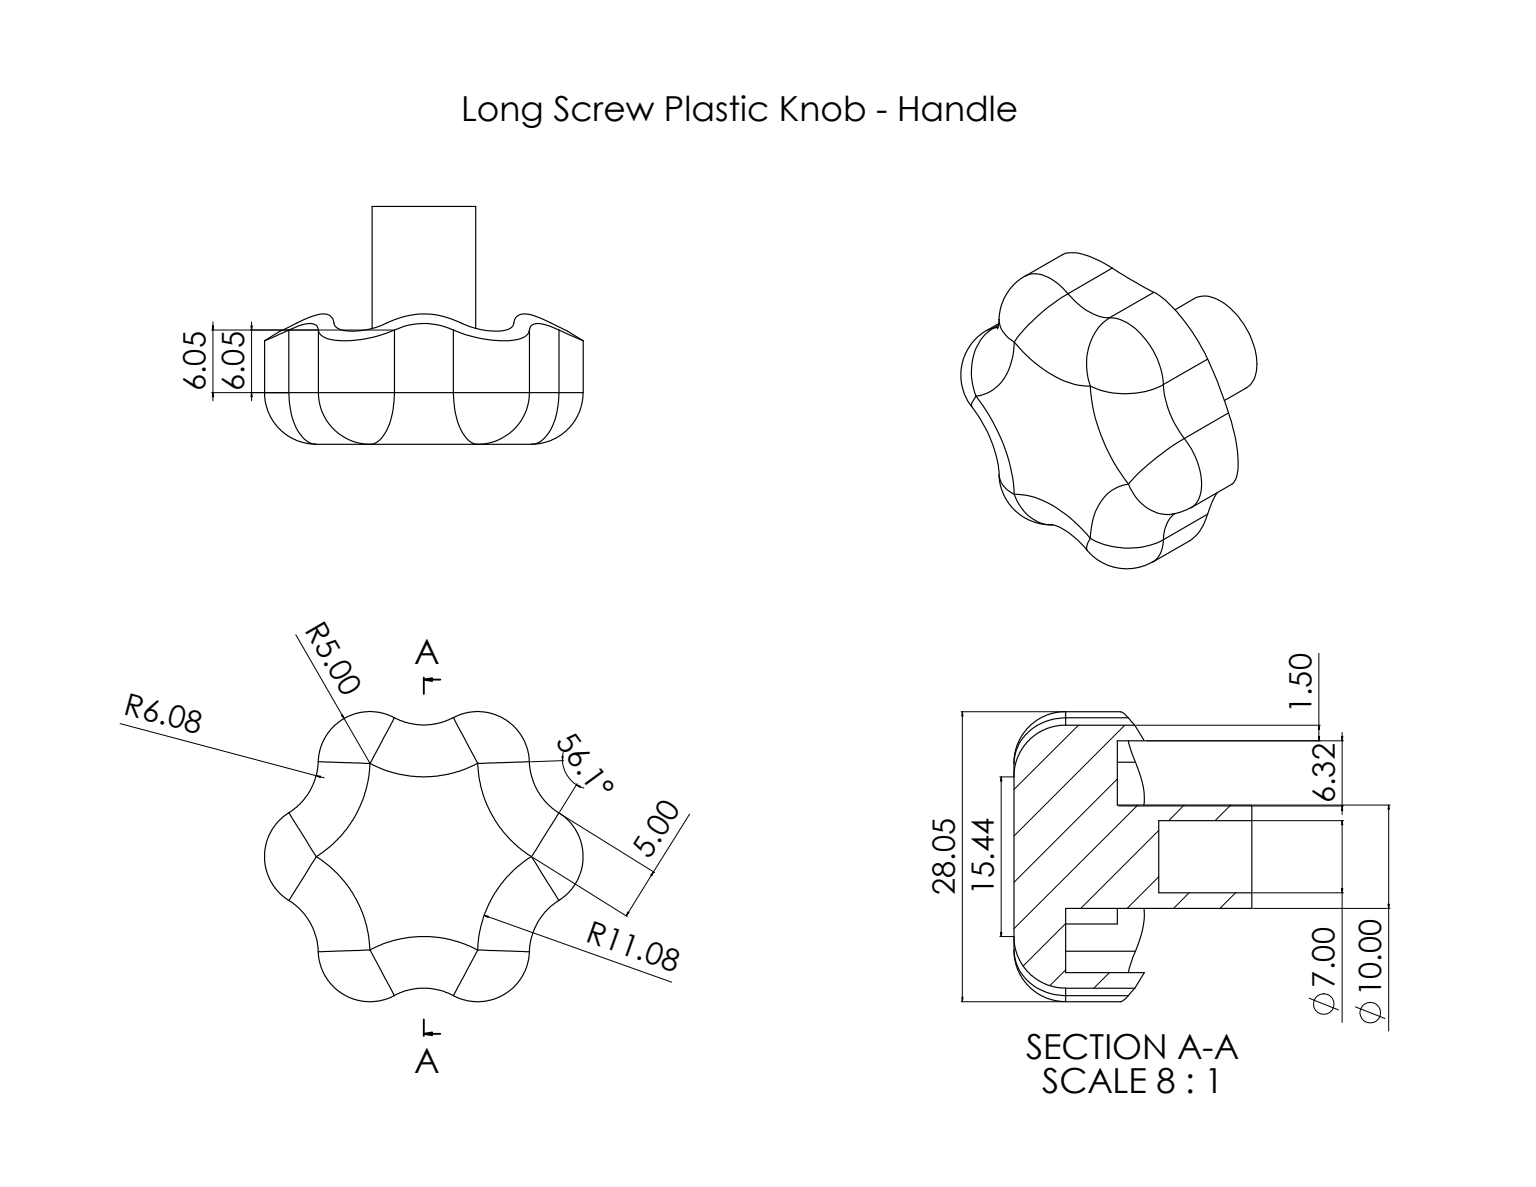
ISO-10303-21;
HEADER;
FILE_DESCRIPTION (('STEP AP214'),
    '1' );
FILE_NAME ('Long Screw Plastic Knob - Handle.step',
    '2026-10-25T21:42:00',
    ( '' ),
    ( '' ),
    'SwSTEP 2.0',
    'SolidWorks 2025',
    '' );
FILE_SCHEMA (( 'AUTOMOTIVE_DESIGN' ));
ENDSEC;

DATA;
#36=CARTESIAN_POINT ( 'NONE',  ( 10.43622283668244677, 12.93305852789453958, 152.0797566693945271 ) ) ;
#58=DIRECTION ( 'NONE',  ( -0.000000000000000000, -0.000000000000000000, -1.000000000000000000 ) ) ;
#59=EDGE_LOOP ( 'NONE', ( #5782, #29938, #317, #14621 ) ) ;
#62=VECTOR ( 'NONE', #37748, 1000.000000000000000 ) ;
#70=DIRECTION ( 'NONE',  ( 0.000000000000000000, 0.000000000000000000, 1.000000000000000000 ) ) ;
#88=CARTESIAN_POINT ( 'NONE',  ( -9.563059451445392156, 11.61997171880338264, 151.9771748954512702 ) ) ;
#133=CARTESIAN_POINT ( 'NONE',  ( -11.30546083962630455, 21.17667637765792676, 152.3877646696492434 ) ) ;
#139=CARTESIAN_POINT ( 'NONE',  ( 12.66061713743917672, 13.00501110736659349, 153.3425884699745723 ) ) ;
#140=CARTESIAN_POINT ( 'NONE',  ( -13.30606428308414380, 19.48475381634399994, 153.3566391844704526 ) ) ;
#160=EDGE_CURVE ( 'NONE', #29981, #18650, #5671, .T. ) ;
#161=CARTESIAN_POINT ( 'NONE',  ( -7.229790860940832786, 5.601750392630878039, 153.6451024802804568 ) ) ;
#162=ORIENTED_EDGE ( 'NONE', *, *, #29231, .F. ) ;
#170=CIRCLE ( 'NONE', #4941, 5.000000000000001776 ) ;
#200=CIRCLE ( 'NONE', #40954, 3.500000000000001332 ) ;
#224=CIRCLE ( 'NONE', #23934, 5.000000000000000888 ) ;
#225=ORIENTED_EDGE ( 'NONE', *, *, #1604, .T. ) ;
#239=CARTESIAN_POINT ( 'NONE',  ( -1.000000000000119460, 22.39897948556632201, 155.5815388724490163 ) ) ;
#242=ADVANCED_FACE ( 'NONE', ( #13025 ), #15594, .T. ) ;
#262=CARTESIAN_POINT ( 'NONE',  ( 12.86284886260855487, 21.86886135845661272, 153.4374325591894603 ) ) ;
#269=DIRECTION ( 'NONE',  ( -0.9994203709764841737, -0.03404294460276034023, 0.000000000000000000 ) ) ;
#299=DIRECTION ( 'NONE',  ( -1.000000000000000000, 0.000000000000000000, 0.000000000000000000 ) ) ;
#311=DIRECTION ( 'NONE',  ( -0.000000000000000000, -0.000000000000000000, -1.000000000000000000 ) ) ;
#313=AXIS2_PLACEMENT_3D ( 'NONE', #32671, #3532, #32264 ) ;
#317=ORIENTED_EDGE ( 'NONE', *, *, #2957, .F. ) ;
#355=CARTESIAN_POINT ( 'NONE',  ( -10.41947860041774199, 17.49999999999951683, 150.5815388724490163 ) ) ;
#361=ORIENTED_EDGE ( 'NONE', *, *, #4016, .F. ) ;
#364=CIRCLE ( 'NONE', #34339, 5.000000000000000888 ) ;
#375=EDGE_CURVE ( 'NONE', #20375, #8168, #5807, .T. ) ;
#378=CARTESIAN_POINT ( 'NONE',  ( -5.521922812467119357, 30.01281927928243221, 153.4949357518731574 ) ) ;
#387=DIRECTION ( 'NONE',  ( 0.000000000000000000, 0.000000000000000000, -1.000000000000000000 ) ) ;
#404=CARTESIAN_POINT ( 'NONE',  ( -5.209739300208506840, 26.52353316214900047, 150.5815388724490163 ) ) ;
#472=ORIENTED_EDGE ( 'NONE', *, *, #35547, .F. ) ;
#481=CARTESIAN_POINT ( 'NONE',  ( -10.21496935922952787, 26.45512302793272497, 153.4374324903474758 ) ) ;
#489=DIRECTION ( 'NONE',  ( -0.000000000000000000, -0.000000000000000000, -1.000000000000000000 ) ) ;
#506=LINE ( 'NONE', #19862, #4090 ) ;
#577=CARTESIAN_POINT ( 'NONE',  ( -2.858598646996059145, 30.93625767528277848, 153.5324451153149710 ) ) ;
#585=CARTESIAN_POINT ( 'NONE',  ( -8.304048588508432971, 28.16586906230009291, 153.3961973886181624 ) ) ;
#594=CARTESIAN_POINT ( 'NONE',  ( -5.000000000000004441, 17.49999999999998934, 159.5815388724490163 ) ) ;
#601=CARTESIAN_POINT ( 'NONE',  ( 3.603329285779394375, 31.27640273042125330, 153.8406024308885947 ) ) ;
#606=CARTESIAN_POINT ( 'NONE',  ( 4.330127018922280691, 15.00000000000012967, 159.5815388724490163 ) ) ;
#610=DIRECTION ( 'NONE',  ( 0.000000000000000000, 0.000000000000000000, -1.000000000000000000 ) ) ;
#624=LINE ( 'NONE', #4028, #9836 ) ;
#640=ORIENTED_EDGE ( 'NONE', *, *, #10319, .F. ) ;
#645=VERTEX_POINT ( 'NONE', #8520 ) ;
#685=EDGE_CURVE ( 'NONE', #37892, #17339, #16571, .T. ) ;
#696=CARTESIAN_POINT ( 'NONE',  ( -11.28839907014780408, 23.42525252760958310, 152.9200731080178457 ) ) ;
#712=EDGE_CURVE ( 'NONE', #26911, #2576, #2299, .T. ) ;
#719=ADVANCED_FACE ( 'NONE', ( #4504 ), #11100, .T. ) ;
#751=ORIENTED_EDGE ( 'NONE', *, *, #36224, .T. ) ;
#782=ADVANCED_FACE ( 'NONE', ( #24490 ), #37459, .T. ) ;
#813=ORIENTED_EDGE ( 'NONE', *, *, #4636, .T. ) ;
#839=CARTESIAN_POINT ( 'NONE',  ( 0.000000000000000000, 17.49999999999998934, 159.5815388724490163 ) ) ;
#841=EDGE_CURVE ( 'NONE', #38078, #4657, #33552, .T. ) ;
#854=CIRCLE ( 'NONE', #40920, 5.000000000000004441 ) ;
#856=ORIENTED_EDGE ( 'NONE', *, *, #19107, .F. ) ;
#859=LINE ( 'NONE', #1078, #3602 ) ;
#908=VECTOR ( 'NONE', #1611, 1000.000000000000000 ) ;
#913=CARTESIAN_POINT ( 'NONE',  ( -10.49927174262155205, 25.01053898198142633, 153.0192155857724572 ) ) ;
#916=CARTESIAN_POINT ( 'NONE',  ( 0.000000000000000000, 17.49999999999998934, 141.5815388724490163 ) ) ;
#919=ORIENTED_EDGE ( 'NONE', *, *, #6532, .F. ) ;
#930=CARTESIAN_POINT ( 'NONE',  ( -1.196959198423996895E-13, 22.49999999999999289, 159.5815388724490163 ) ) ;
#973=DIRECTION ( 'NONE',  ( 1.000000000000000000, 0.000000000000000000, 0.000000000000000000 ) ) ;
#984=DIRECTION ( 'NONE',  ( -0.000000000000000000, -0.000000000000000000, -1.000000000000000000 ) ) ;
#990=LINE ( 'NONE', #39688, #24682 ) ;
#1007=AXIS2_PLACEMENT_3D ( 'NONE', #15270, #22266, #9511 ) ;
#1046=CYLINDRICAL_SURFACE ( 'NONE', #23464, 5.000000000000000000 ) ;
#1050=DIRECTION ( 'NONE',  ( 0.5291922403339774927, -0.8485019580238492010, 0.000000000000000000 ) ) ;
#1078=CARTESIAN_POINT ( 'NONE',  ( 1.000000000000119460, 5.911571776152701574, 154.5815388724490163 ) ) ;
#1114=DIRECTION ( 'NONE',  ( -1.000000000000000000, 0.000000000000000000, 0.000000000000000000 ) ) ;
#1129=AXIS2_PLACEMENT_3D ( 'NONE', #24829, #30991, #12470 ) ;
#1153=CARTESIAN_POINT ( 'NONE',  ( -10.49712838360467160, 9.983023053045442907, 153.0204462789266131 ) ) ;
#1168=VERTEX_POINT ( 'NONE', #3968 ) ;
#1178=CARTESIAN_POINT ( 'NONE',  ( -10.20684115509089729, 26.69374788516367758, 159.5815388724490163 ) ) ;
#1181=CARTESIAN_POINT ( 'NONE',  ( 0.000000000000000000, 17.49999999999956302, 154.9135024962512546 ) ) ;
#1197=DIRECTION ( 'NONE',  ( 0.000000000000000000, 0.000000000000000000, 1.000000000000000000 ) ) ;
#1230=ORIENTED_EDGE ( 'NONE', *, *, #21514, .F. ) ;
#1233=( NAMED_UNIT ( * ) SI_UNIT ( $, .STERADIAN. ) SOLID_ANGLE_UNIT ( ) );
#1237=ORIENTED_EDGE ( 'NONE', *, *, #40727, .F. ) ;
#1247=LINE ( 'NONE', #11028, #6038 ) ;
#1277=EDGE_CURVE ( 'NONE', #3405, #3157, #40350, .T. ) ;
#1315=DIRECTION ( 'NONE',  ( -0.000000000000000000, 0.000000000000000000, 1.000000000000000000 ) ) ;
#1319=CARTESIAN_POINT ( 'NONE',  ( -10.03587323178440194, 23.29421411192350178, 154.5815388724490163 ) ) ;
#1323=ORIENTED_EDGE ( 'NONE', *, *, #13033, .T. ) ;
#1359=CARTESIAN_POINT ( 'NONE',  ( -10.22308315533814316, 8.783078843579193773, 153.3425882844790067 ) ) ;
#1372=CARTESIAN_POINT ( 'NONE',  ( -2.858598646996156400, 4.063742324715559739, 153.5324451153154541 ) ) ;
#1439=FACE_OUTER_BOUND ( 'NONE', #37211, .T. ) ;
#1444=B_SPLINE_CURVE_WITH_KNOTS ( 'NONE', 3,
 ( #38980, #35787, #33219, #36634, #13036, #3662, #29392, #19825, #20048, #10688, #7286, #20256, #23671, #17068, #262, #26227 ),
 .UNSPECIFIED., .F., .F.,
 ( 4, 2, 2, 2, 2, 2, 2, 4 ),
 ( 2.129600427422370939E-07, 0.001523388048537042310, 0.002284975592784182705, 0.003046563137031323316, 0.003808150681278463495, 0.004569738225525604540, 0.005331325769772745152, 0.006092913314019885763 ),
 .UNSPECIFIED. ) ;
#1464=CARTESIAN_POINT ( 'NONE',  ( 10.41947860041720908, 17.49999999999956302, 159.5815388724490163 ) ) ;
#1516=CARTESIAN_POINT ( 'NONE',  ( 5.209739300208926949, 8.476466837849169877, 159.5815388724490163 ) ) ;
#1523=CARTESIAN_POINT ( 'NONE',  ( 16.28249153430138207, 8.099299129593287461, 159.5815388724490163 ) ) ;
#1531=CARTESIAN_POINT ( 'NONE',  ( 7.470466625468908717, 29.21249557649308670, 153.6264001176285205 ) ) ;
#1534=DIRECTION ( 'NONE',  ( -1.000000000000000000, 0.000000000000000000, 0.000000000000000000 ) ) ;
#1542=CARTESIAN_POINT ( 'NONE',  ( 16.28249153430138207, 8.099299129593287461, 154.5815388724490163 ) ) ;
#1575=ORIENTED_EDGE ( 'NONE', *, *, #40939, .T. ) ;
#1592=CARTESIAN_POINT ( 'NONE',  ( 0.000000000000000000, 17.49999999999998934, 159.5815388724490163 ) ) ;
#1604=EDGE_CURVE ( 'NONE', #13562, #20191, #10047, .T. ) ;
#1609=DIRECTION ( 'NONE',  ( -0.000000000000000000, -0.000000000000000000, 1.000000000000000000 ) ) ;
#1611=DIRECTION ( 'NONE',  ( -0.000000000000000000, -0.000000000000000000, -1.000000000000000000 ) ) ;
#1623=VERTEX_POINT ( 'NONE', #13865 ) ;
#1633=ORIENTED_EDGE ( 'NONE', *, *, #40040, .F. ) ;
#1672=ORIENTED_EDGE ( 'NONE', *, *, #15832, .T. ) ;
#1682=CARTESIAN_POINT ( 'NONE',  ( -16.28249153430137497, 8.099299129593275026, 154.5815388724490163 ) ) ;
#1693=EDGE_CURVE ( 'NONE', #14205, #23076, #12143, .T. ) ;
#1698=VECTOR ( 'NONE', #15687, 1000.000000000000000 ) ;
#1716=CONICAL_SURFACE ( 'NONE', #40427, 15.97057991159785217, 1.017022292416746465 ) ;
#1733=CARTESIAN_POINT ( 'NONE',  ( 9.883105000805365137, 22.82715757353904351, 151.9779334031984774 ) ) ;
#1738=CARTESIAN_POINT ( 'NONE',  ( 0.000000000000000000, 36.30140174081339666, 159.5815388724490163 ) ) ;
#1741=ORIENTED_EDGE ( 'NONE', *, *, #40653, .F. ) ;
#1751=EDGE_CURVE ( 'NONE', #7452, #37682, #14909, .T. ) ;
#1771=CARTESIAN_POINT ( 'NONE',  ( 0.000000000000000000, 0.000000000000000000, 150.5815388724490163 ) ) ;
#1772=CARTESIAN_POINT ( 'NONE',  ( -2.858598646996156400, 4.063742324715559739, 153.5324451153154541 ) ) ;
#1780=ORIENTED_EDGE ( 'NONE', *, *, #10909, .T. ) ;
#1782=ADVANCED_FACE ( 'NONE', ( #8938 ), #5025, .T. ) ;
#1785=EDGE_CURVE ( 'NONE', #32027, #13358, #24912, .T. ) ;
#1788=CARTESIAN_POINT ( 'NONE',  ( -1.974753549813219378, 4.453261797671114408, 153.1965160626535578 ) ) ;
#1816=CARTESIAN_POINT ( 'NONE',  ( 3.500000000000003997, 17.49999999999998934, 155.5815388724490163 ) ) ;
#1834=CARTESIAN_POINT ( 'NONE',  ( -15.41947860041774376, 17.49999999999956657, 154.5727510624246293 ) ) ;
#1852=CARTESIAN_POINT ( 'NONE',  ( -14.54815605848680171, 20.32812363823408575, 154.2016373142952830 ) ) ;
#1859=ORIENTED_EDGE ( 'NONE', *, *, #24561, .F. ) ;
#1864=CARTESIAN_POINT ( 'NONE',  ( -9.718734271692440529, 11.88888615205571320, 159.5815388724490163 ) ) ;
#1875=ORIENTED_EDGE ( 'NONE', *, *, #15991, .T. ) ;
#1878=DIRECTION ( 'NONE',  ( 1.000000000000000000, 0.000000000000000000, 0.000000000000000000 ) ) ;
#1899=VERTEX_POINT ( 'NONE', #31694 ) ;
#1910=CARTESIAN_POINT ( 'NONE',  ( 8.534991945851601258, 7.374913356028258704, 153.2263581680556115 ) ) ;
#1929=DIRECTION ( 'NONE',  ( -0.000000000000000000, 0.000000000000000000, 1.000000000000000000 ) ) ;
#1941=CARTESIAN_POINT ( 'NONE',  ( -1.196959198423996895E-13, 29.08842822384727356, 159.5815388724490163 ) ) ;
#1954=ORIENTED_EDGE ( 'NONE', *, *, #1785, .F. ) ;
#1992=ORIENTED_EDGE ( 'NONE', *, *, #19993, .F. ) ;
#2041=VECTOR ( 'NONE', #21924, 1000.000000000000000 ) ;
#2042=ORIENTED_EDGE ( 'NONE', *, *, #16249, .F. ) ;
#2056=DIRECTION ( 'NONE',  ( -0.8660254037844432595, 0.4999999999999919509, 0.000000000000000000 ) ) ;
#2068=DIRECTION ( 'NONE',  ( 0.000000000000000000, 0.000000000000000000, -1.000000000000000000 ) ) ;
#2076=CARTESIAN_POINT ( 'NONE',  ( 0.000000000000000000, 17.49999999999998934, 159.5815388724490163 ) ) ;
#2081=DIRECTION ( 'NONE',  ( -0.8660254037844432595, 0.4999999999999918954, 0.000000000000000000 ) ) ;
#2094=VERTEX_POINT ( 'NONE', #13822 ) ;
#2098=ORIENTED_EDGE ( 'NONE', *, *, #3993, .F. ) ;
#2101=DIRECTION ( 'NONE',  ( 1.000000000000000000, 0.000000000000000000, 0.000000000000000000 ) ) ;
#2105=DIRECTION ( 'NONE',  ( 1.000000000000000000, 3.562084945903540364E-15, 0.000000000000000000 ) ) ;
#2106=ORIENTED_EDGE ( 'NONE', *, *, #16512, .T. ) ;
#2146=ORIENTED_EDGE ( 'NONE', *, *, #27392, .T. ) ;
#2170=AXIS2_PLACEMENT_3D ( 'NONE', #32736, #7869, #33377 ) ;
#2193=EDGE_CURVE ( 'NONE', #15661, #40121, #624, .T. ) ;
#2209=ORIENTED_EDGE ( 'NONE', *, *, #18837, .F. ) ;
#2212=CARTESIAN_POINT ( 'NONE',  ( 12.73537588372913554, 20.13994587915788870, 153.0791759260050355 ) ) ;
#2257=VERTEX_POINT ( 'NONE', #23096 ) ;
#2272=CARTESIAN_POINT ( 'NONE',  ( -14.16111231062272324, 14.17694842453450299, 154.0318591658869138 ) ) ;
#2284=LINE ( 'NONE', #11847, #10538 ) ;
#2299=CIRCLE ( 'NONE', #36958, 7.579174044925481191 ) ;
#2302=CARTESIAN_POINT ( 'NONE',  ( 10.53587323178443569, 12.57181129186098723, 154.5815388724490163 ) ) ;
#2308=EDGE_CURVE ( 'NONE', #10845, #10531, #16114, .T. ) ;
#2311=ADVANCED_FACE ( 'NONE', ( #35660 ), #2322, .T. ) ;
#2322=CONICAL_SURFACE ( 'NONE', #38330, 15.97057991159785217, 1.017022292416746465 ) ;
#2337=CARTESIAN_POINT ( 'NONE',  ( 8.304048588509031603, 6.834130937698395414, 153.3961973886187025 ) ) ;
#2377=ORIENTED_EDGE ( 'NONE', *, *, #32906, .T. ) ;
#2421=ORIENTED_EDGE ( 'NONE', *, *, #34771, .T. ) ;
#2468=ORIENTED_EDGE ( 'NONE', *, *, #13201, .F. ) ;
#2489=VERTEX_POINT ( 'NONE', #29953 ) ;
#2492=FACE_OUTER_BOUND ( 'NONE', #42089, .T. ) ;
#2493=DIRECTION ( 'NONE',  ( -0.000000000000000000, -0.000000000000000000, -1.000000000000000000 ) ) ;
#2515=CARTESIAN_POINT ( 'NONE',  ( -12.27165144158654542, 14.53024314691596963, 152.8454421597759563 ) ) ;
#2523=ORIENTED_EDGE ( 'NONE', *, *, #39714, .T. ) ;
#2564=ORIENTED_EDGE ( 'NONE', *, *, #29829, .F. ) ;
#2576=VERTEX_POINT ( 'NONE', #30380 ) ;
#2578=PLANE ( 'NONE',  #26237 ) ;
#2600=CARTESIAN_POINT ( 'NONE',  ( 15.12727392775252966, 15.80214688207034968, 154.4499356296060739 ) ) ;
#2603=DIRECTION ( 'NONE',  ( 0.8660254037844432595, -0.4999999999999919509, 0.000000000000000000 ) ) ;
#2604=ADVANCED_FACE ( 'NONE', ( #14845 ), #4848, .T. ) ;
#2608=DIRECTION ( 'NONE',  ( 0.000000000000000000, 0.000000000000000000, 1.000000000000000000 ) ) ;
#2631=DIRECTION ( 'NONE',  ( -0.000000000000000000, 0.000000000000000000, 1.000000000000000000 ) ) ;
#2638=CARTESIAN_POINT ( 'NONE',  ( 3.563940842959628874, 29.61244032134256088, 159.5815388724490163 ) ) ;
#2653=ADVANCED_FACE ( 'NONE', ( #37189 ), #6422, .T. ) ;
#2670=CARTESIAN_POINT ( 'NONE',  ( 1.000000000000119460, 12.60102051443365134, 159.5815388724490163 ) ) ;
#2682=VERTEX_POINT ( 'NONE', #7628 ) ;
#2689=CARTESIAN_POINT ( 'NONE',  ( -15.41947860041774909, 17.06357649946066601, 154.5727510624246861 ) ) ;
#2727=CARTESIAN_POINT ( 'NONE',  ( -3.563940842960075184, 5.387559678655594375, 152.8454421597761552 ) ) ;
#2731=CARTESIAN_POINT ( 'NONE',  ( -1.268010732602997237, 6.177570447869829451, 152.0807008677966223 ) ) ;
#2742=ORIENTED_EDGE ( 'NONE', *, *, #13033, .F. ) ;
#2744=EDGE_CURVE ( 'NONE', #41665, #32078, #27610, .T. ) ;
#2754=CIRCLE ( 'NONE', #26549, 4.999999999999999112 ) ;
#2770=DIRECTION ( 'NONE',  ( -0.000000000000000000, -0.000000000000000000, -1.000000000000000000 ) ) ;
#2798=VERTEX_POINT ( 'NONE', #14017 ) ;
#2816=CARTESIAN_POINT ( 'NONE',  ( 15.41947860041720553, 17.06271552903863054, 154.5727510624243166 ) ) ;
#2859=CIRCLE ( 'NONE', #8288, 5.000000000000004441 ) ;
#2880=CIRCLE ( 'NONE', #22575, 5.000000000000004441 ) ;
#2883=AXIS2_PLACEMENT_3D ( 'NONE', #41231, #9102, #22082 ) ;
#2893=ORIENTED_EDGE ( 'NONE', *, *, #6437, .T. ) ;
#2912=UNCERTAINTY_MEASURE_WITH_UNIT (LENGTH_MEASURE( 1.000000000000000082E-05 ), #13359, 'distance_accuracy_value', 'NONE');
#2915=CARTESIAN_POINT ( 'NONE',  ( -9.555006584822248072, 23.39544065986577692, 151.9779333824603214 ) ) ;
#2925=DIRECTION ( 'NONE',  ( 0.000000000000000000, 0.000000000000000000, -1.000000000000000000 ) ) ;
#2941=CARTESIAN_POINT ( 'NONE',  ( -8.654913651898935356, 7.795446523357140833, 153.0774312600626956 ) ) ;
#2943=CARTESIAN_POINT ( 'NONE',  ( -7.786277848952735781, 28.89725529122591041, 153.5727845928841191 ) ) ;
#2955=ORIENTED_EDGE ( 'NONE', *, *, #40653, .T. ) ;
#2956=EDGE_CURVE ( 'NONE', #28523, #29981, #38995, .T. ) ;
#2957=EDGE_CURVE ( 'NONE', #3492, #4147, #19324, .T. ) ;
#2959=CARTESIAN_POINT ( 'NONE',  ( 4.204107165319143746, 31.42570457654730731, 154.0322825799475766 ) ) ;
#2981=ORIENTED_EDGE ( 'NONE', *, *, #25435, .T. ) ;
#2998=ORIENTED_EDGE ( 'NONE', *, *, #30412, .F. ) ;
#3010=ADVANCED_FACE ( 'NONE', ( #25474 ), #9301, .F. ) ;
#3016=CARTESIAN_POINT ( 'NONE',  ( 5.209739300208269697, 26.52353316214887613, 159.5815388724490163 ) ) ;
#3023=CARTESIAN_POINT ( 'NONE',  ( 15.41947860041720908, 17.49999999999956302, 154.5727510624243166 ) ) ;
#3049=FACE_OUTER_BOUND ( 'NONE', #26591, .T. ) ;
#3061=AXIS2_PLACEMENT_3D ( 'NONE', #11887, #24879, #37839 ) ;
#3071=ADVANCED_FACE ( 'NONE', ( #39689 ), #23542, .F. ) ;
#3095=DIRECTION ( 'NONE',  ( -1.000000000000000000, 0.000000000000000000, 0.000000000000000000 ) ) ;
#3112=CARTESIAN_POINT ( 'NONE',  ( -10.41947860041774199, 17.49999999999951683, 159.5815388724490163 ) ) ;
#3129=CARTESIAN_POINT ( 'NONE',  ( -11.07557039803294607, 21.38447842288499601, 152.2937014864026537 ) ) ;
#3156=CARTESIAN_POINT ( 'NONE',  ( -8.536601555666415209, 7.379771219736498189, 153.2247034666974912 ) ) ;
#3157=VERTEX_POINT ( 'NONE', #29905 ) ;
#3205=EDGE_LOOP ( 'NONE', ( #17899, #20292, #4413 ) ) ;
#3241=ORIENTED_EDGE ( 'NONE', *, *, #32380, .F. ) ;
#3257=ORIENTED_EDGE ( 'NONE', *, *, #33128, .T. ) ;
#3259=CARTESIAN_POINT ( 'NONE',  ( 10.41947860041720908, 17.49999999999956302, 159.5815388724490163 ) ) ;
#3286=CARTESIAN_POINT ( 'NONE',  ( -9.173198941869365797, 10.74543714401176864, 152.0797565808659897 ) ) ;
#3338=DIRECTION ( 'NONE',  ( 0.000000000000000000, 0.000000000000000000, 1.000000000000000000 ) ) ;
#3360=CARTESIAN_POINT ( 'NONE',  ( 0.6437596841449632068, 28.74306530438873963, 151.9992204069320962 ) ) ;
#3361=ORIENTED_EDGE ( 'NONE', *, *, #32867, .F. ) ;
#3362=CARTESIAN_POINT ( 'NONE',  ( 13.06543980208692446, 21.74250979011891971, 150.5815388724490163 ) ) ;
#3373=AXIS2_PLACEMENT_3D ( 'NONE', #38028, #27624, #20833 ) ;
#3377=CIRCLE ( 'NONE', #31912, 5.000000000000004441 ) ;
#3379=CARTESIAN_POINT ( 'NONE',  ( 6.938007057734065341, 31.23522659030811610, 154.5496812852157404 ) ) ;
#3387=CARTESIAN_POINT ( 'NONE',  ( -2.858598646996158177, 4.063742324715557963, 159.5815388724490163 ) ) ;
#3405=VERTEX_POINT ( 'NONE', #28327 ) ;
#3429=AXIS2_PLACEMENT_3D ( 'NONE', #31143, #2631, #25401 ) ;
#3432=CARTESIAN_POINT ( 'NONE',  ( 10.64084095417626230, 13.17005021218726135, 152.1397378211943590 ) ) ;
#3452=DIRECTION ( 'NONE',  ( -1.000000000000000000, 0.000000000000000000, 0.000000000000000000 ) ) ;
#3492=VERTEX_POINT ( 'NONE', #6205 ) ;
#3510=DIRECTION ( 'NONE',  ( -0.8660254037844328234, -0.5000000000000101030, 0.000000000000000000 ) ) ;
#3532=DIRECTION ( 'NONE',  ( 0.000000000000000000, 0.000000000000000000, 1.000000000000000000 ) ) ;
#3558=CARTESIAN_POINT ( 'NONE',  ( -5.084889071861075749, 4.975548446798801372, 153.3961973379654182 ) ) ;
#3564=VERTEX_POINT ( 'NONE', #23199 ) ;
#3577=CARTESIAN_POINT ( 'NONE',  ( 2.302507646137074410E-15, -1.301401740813418195, 154.5815388724490163 ) ) ;
#3602=VECTOR ( 'NONE', #36804, 1000.000000000000000 ) ;
#3603=CARTESIAN_POINT ( 'NONE',  ( -2.858598646996059145, 30.93625767528277848, 153.5324451153149710 ) ) ;
#3607=ORIENTED_EDGE ( 'NONE', *, *, #24128, .T. ) ;
#3612=ORIENTED_EDGE ( 'NONE', *, *, #11547, .T. ) ;
#3653=VECTOR ( 'NONE', #14292, 1000.000000000000114 ) ;
#3662=CARTESIAN_POINT ( 'NONE',  ( 10.77561899351920793, 24.31341356600224302, 152.9200730590035846 ) ) ;
#3676=EDGE_CURVE ( 'NONE', #26392, #16970, #31556, .T. ) ;
#3702=ORIENTED_EDGE ( 'NONE', *, *, #27531, .F. ) ;
#3719=AXIS2_PLACEMENT_3D ( 'NONE', #916, #7508, #33021 ) ;
#3720=DIRECTION ( 'NONE',  ( -0.000000000000000000, -0.000000000000000000, -1.000000000000000000 ) ) ;
#3750=CARTESIAN_POINT ( 'NONE',  ( 14.29598715238342699, 20.66495239839645137, 154.0913466422284728 ) ) ;
#3751=CARTESIAN_POINT ( 'NONE',  ( -13.91947860041774021, 17.80787983862214219, 153.6452861111158086 ) ) ;
#3772=ORIENTED_EDGE ( 'NONE', *, *, #11377, .F. ) ;
#3794=CARTESIAN_POINT ( 'NONE',  ( 3.217162522966638960, 31.12730384257888971, 153.6941203706221870 ) ) ;
#3800=DIRECTION ( 'NONE',  ( -0.000000000000000000, -0.000000000000000000, -1.000000000000000000 ) ) ;
#3805=DIRECTION ( 'NONE',  ( 0.000000000000000000, 0.000000000000000000, -1.000000000000000000 ) ) ;
#3835=EDGE_CURVE ( 'NONE', #2257, #6594, #36327, .T. ) ;
#3854=EDGE_CURVE ( 'NONE', #28523, #29783, #34292, .T. ) ;
#3864=CARTESIAN_POINT ( 'NONE',  ( -6.938007057734935756, 3.764773409689712302, 154.5496812852166784 ) ) ;
#3871=CARTESIAN_POINT ( 'NONE',  ( 5.827333669638361968, 29.97187497973753878, 153.5499869721883783 ) ) ;
#3923=CARTESIAN_POINT ( 'NONE',  ( -13.12951721863655585, 15.28026294324127576, 153.2716563237898697 ) ) ;
#3961=CARTESIAN_POINT ( 'NONE',  ( 10.21496935922993288, 8.544876972066248300, 153.4374324903477600 ) ) ;
#3962=LINE ( 'NONE', #13532, #26130 ) ;
#3968=CARTESIAN_POINT ( 'NONE',  ( 9.276117013689805901, 24.01026919326780629, 159.5815388724490163 ) ) ;
#3993=EDGE_CURVE ( 'NONE', #2576, #8117, #12535, .T. ) ;
#4013=DIRECTION ( 'NONE',  ( -1.000000000000000000, 0.000000000000000000, 0.000000000000000000 ) ) ;
#4016=EDGE_CURVE ( 'NONE', #8962, #38078, #35504, .T. ) ;
#4028=CARTESIAN_POINT ( 'NONE',  ( 10.03587323178444279, 11.70578588807654441, 154.5815388724490163 ) ) ;
#4035=ORIENTED_EDGE ( 'NONE', *, *, #32928, .F. ) ;
#4077=DIRECTION ( 'NONE',  ( -0.000000000000000000, -0.000000000000000000, -1.000000000000000000 ) ) ;
#4090=VECTOR ( 'NONE', #39013, 1000.000000000000000 ) ;
#4094=CARTESIAN_POINT ( 'NONE',  ( 3.500000000000003997, 17.49999999999998934, 150.5815388724490163 ) ) ;
#4147=VERTEX_POINT ( 'NONE', #16784 ) ;
#4152=VECTOR ( 'NONE', #15554, 1000.000000000000000 ) ;
#4173=CARTESIAN_POINT ( 'NONE',  ( -4.330127018922262927, 19.99999999999987566, 155.5815388724490163 ) ) ;
#4182=CARTESIAN_POINT ( 'NONE',  ( 5.209739300208269697, 26.52353316214887613, 159.5815388724490163 ) ) ;
#4183=ORIENTED_EDGE ( 'NONE', *, *, #4675, .T. ) ;
#4197=ORIENTED_EDGE ( 'NONE', *, *, #26666, .F. ) ;
#4206=AXIS2_PLACEMENT_3D ( 'NONE', #35238, #36711, #10561 ) ;
#4225=CARTESIAN_POINT ( 'NONE',  ( 5.209739300208926061, 8.476466837849169877, 150.5815388724490163 ) ) ;
#4232=DIRECTION ( 'NONE',  ( 0.5000000000000039968, -0.8660254037844363761, 0.000000000000000000 ) ) ;
#4244=DIRECTION ( 'NONE',  ( -1.000000000000000000, 0.000000000000000000, -0.000000000000000000 ) ) ;
#4245=ORIENTED_EDGE ( 'NONE', *, *, #9976, .T. ) ;
#4247=TOROIDAL_SURFACE ( 'NONE', #23961, 11.07917404492595814, 5.000000000000000000 ) ;
#4252=ORIENTED_EDGE ( 'NONE', *, *, #24650, .T. ) ;
#4257=ADVANCED_FACE ( 'NONE', ( #7212 ), #1046, .T. ) ;
#4262=VERTEX_POINT ( 'NONE', #606 ) ;
#4269=VECTOR ( 'NONE', #37406, 1000.000000000000000 ) ;
#4295=CARTESIAN_POINT ( 'NONE',  ( 10.41947860041720908, 17.49999999999956302, 150.5815388724490163 ) ) ;
#4308=ORIENTED_EDGE ( 'NONE', *, *, #9976, .F. ) ;
#4334=DIRECTION ( 'NONE',  ( -0.000000000000000000, -0.000000000000000000, -1.000000000000000000 ) ) ;
#4336=DIRECTION ( 'NONE',  ( -1.000000000000000000, 0.000000000000000000, 0.000000000000000000 ) ) ;
#4340=ORIENTED_EDGE ( 'NONE', *, *, #40701, .T. ) ;
#4343=AXIS2_PLACEMENT_3D ( 'NONE', #19268, #3720, #25661 ) ;
#4363=DIRECTION ( 'NONE',  ( 0.000000000000000000, 0.000000000000000000, 1.000000000000000000 ) ) ;
#4399=VERTEX_POINT ( 'NONE', #36268 ) ;
#4413=ORIENTED_EDGE ( 'NONE', *, *, #20722, .T. ) ;
#4416=CARTESIAN_POINT ( 'NONE',  ( -8.707710598626182019, 26.64268346825927836, 152.8454421597756436 ) ) ;
#4429=AXIS2_PLACEMENT_3D ( 'NONE', #39570, #7255, #20227 ) ;
#4434=ADVANCED_FACE ( 'NONE', ( #33286 ), #1716, .T. ) ;
#4470=VERTEX_POINT ( 'NONE', #23947 ) ;
#4502=CARTESIAN_POINT ( 'NONE',  ( -4.204107165319530992, 3.574295423450687625, 154.0322825799484008 ) ) ;
#4504=FACE_OUTER_BOUND ( 'NONE', #41210, .T. ) ;
#4507=CARTESIAN_POINT ( 'NONE',  ( 11.77029632476400245, 20.78244114917104568, 152.5896212872837054 ) ) ;
#4508=CARTESIAN_POINT ( 'NONE',  ( 6.697448051447455697, 29.70650749756346798, 153.6454670853904929 ) ) ;
#4520=CARTESIAN_POINT ( 'NONE',  ( -10.89329215898964698, 24.07621678493666906, 152.9047840745570568 ) ) ;
#4522=( GEOMETRIC_REPRESENTATION_CONTEXT ( 3 ) GLOBAL_UNCERTAINTY_ASSIGNED_CONTEXT ( ( #2912 ) ) GLOBAL_UNIT_ASSIGNED_CONTEXT ( ( #13359, #34175, #1233 ) ) REPRESENTATION_CONTEXT ( 'NONE', 'WORKASPACE' ) );
#4556=B_SPLINE_CURVE_WITH_KNOTS ( 'NONE', 3,
 ( #22498, #15712, #2941, #3156, #25706, #6126, #32072, #38879, #18893, #29289, #15930, #16345, #161, #9540, #16146, #29084, #25498, #38669, #12936, #3558, #35482, #19523, #42082, #25916, #9755, #2727 ),
 .UNSPECIFIED., .F., .F.,
 ( 4, 2, 2, 2, 2, 2, 2, 2, 2, 2, 2, 2, 4 ),
 ( 2.152236452720500467E-07, 0.0009105534912597466760, 0.001365722625066985137, 0.001820891758874223706, 0.002276060892681462059, 0.002731230026488700845, 0.003641568294103180153, 0.004551906561717659026, 0.005007075695524905619, 0.005462244829332150477, 0.005917413963139396202, 0.006372583096946641060, 0.007282921364561104755 ),
 .UNSPECIFIED. ) ;
#4557=CARTESIAN_POINT ( 'NONE',  ( -3.500000000000003997, 17.49999999999998934, 150.5815388724490163 ) ) ;
#4585=B_SPLINE_CURVE_WITH_KNOTS ( 'NONE', 3,
 ( #24866, #8682, #30822, #40397, #15294, #3360, #28879, #35266, #32289, #5920, #22291, #38462, #19106, #41876, #12727, #12295 ),
 .UNSPECIFIED., .F., .F.,
 ( 4, 2, 2, 2, 2, 2, 2, 4 ),
 ( 2.442785351375339512E-07, 0.001910986702701202066, 0.002866357914784243080, 0.003821729126867285178, 0.004777100338950327277, 0.005732471551033368508, 0.006687842763116409739, 0.007643213975199451837 ),
 .UNSPECIFIED. ) ;
#4612=FACE_OUTER_BOUND ( 'NONE', #3205, .T. ) ;
#4616=ORIENTED_EDGE ( 'NONE', *, *, #17565, .T. ) ;
#4630=ADVANCED_FACE ( 'NONE', ( #27745 ), #30947, .T. ) ;
#4635=CARTESIAN_POINT ( 'NONE',  ( -4.742640687119331844, 19.08346433899860273, 155.5815388724490163 ) ) ;
#4636=EDGE_CURVE ( 'NONE', #33258, #26911, #21417, .T. ) ;
#4638=LINE ( 'NONE', #17616, #28163 ) ;
#4657=VERTEX_POINT ( 'NONE', #5407 ) ;
#4671=VERTEX_POINT ( 'NONE', #8183 ) ;
#4675=EDGE_CURVE ( 'NONE', #2798, #26392, #41812, .T. ) ;
#4683=ORIENTED_EDGE ( 'NONE', *, *, #34455, .T. ) ;
#4691=DIRECTION ( 'NONE',  ( 1.000000000000000000, 0.000000000000000000, 0.000000000000000000 ) ) ;
#4713=CARTESIAN_POINT ( 'NONE',  ( 8.745125217306711107, 26.05017165142009361, 152.5993402266560679 ) ) ;
#4718=CARTESIAN_POINT ( 'NONE',  ( 8.075457743340587413, 28.53853537488712888, 153.4949358233095325 ) ) ;
#4754=CARTESIAN_POINT ( 'NONE',  ( -10.88765427151144571, 10.91299973181360450, 152.9052493511311468 ) ) ;
#4779=ORIENTED_EDGE ( 'NONE', *, *, #15832, .F. ) ;
#4839=VECTOR ( 'NONE', #20542, 1000.000000000000000 ) ;
#4845=DIRECTION ( 'NONE',  ( -0.8660254037844328234, -0.5000000000000101030, 0.000000000000000000 ) ) ;
#4848=CYLINDRICAL_SURFACE ( 'NONE', #12525, 5.000000000000004441 ) ;
#4862=DIRECTION ( 'NONE',  ( 0.000000000000000000, 1.000000000000000000, 0.000000000000000000 ) ) ;
#4873=ORIENTED_EDGE ( 'NONE', *, *, #13006, .F. ) ;
#4874=CARTESIAN_POINT ( 'NONE',  ( -8.707710598626928089, 8.357316531739311216, 159.5815388724490163 ) ) ;
#4941=AXIS2_PLACEMENT_3D ( 'NONE', #24828, #12251, #25236 ) ;
#4966=DIRECTION ( 'NONE',  ( 0.000000000000000000, 1.000000000000000000, 0.000000000000000000 ) ) ;
#4969=DIRECTION ( 'NONE',  ( 0.000000000000000000, 1.000000000000000000, 0.000000000000000000 ) ) ;
#4973=AXIS2_PLACEMENT_3D ( 'NONE', #8074, #31242, #2105 ) ;
#5025=TOROIDAL_SURFACE ( 'NONE', #10467, 11.07917404492548030, 5.000000000000000000 ) ;
#5032=EDGE_LOOP ( 'NONE', ( #24242, #41500, #5467, #26629 ) ) ;
#5070=VECTOR ( 'NONE', #19222, 1000.000000000000000 ) ;
#5080=ORIENTED_EDGE ( 'NONE', *, *, #15741, .F. ) ;
#5089=CIRCLE ( 'NONE', #7135, 5.000000000000000000 ) ;
#5112=CARTESIAN_POINT ( 'NONE',  ( 11.77722871187724252, 14.20158540853836193, 152.5993403437909706 ) ) ;
#5127=AXIS2_PLACEMENT_3D ( 'NONE', #25479, #12062, #6105 ) ;
#5139=DIRECTION ( 'NONE',  ( -0.000000000000000000, 0.000000000000000000, 1.000000000000000000 ) ) ;
#5140=EDGE_CURVE ( 'NONE', #29783, #20414, #32700, .T. ) ;
#5170=DIRECTION ( 'NONE',  ( -0.000000000000000000, 0.000000000000000000, 1.000000000000000000 ) ) ;
#5183=CARTESIAN_POINT ( 'NONE',  ( 9.535873231784194104, 24.16023951570828032, 154.5815388724490163 ) ) ;
#5184=CARTESIAN_POINT ( 'NONE',  ( 7.326644855052992789, 3.925684524727749647, 154.5725613197538735 ) ) ;
#5194=VERTEX_POINT ( 'NONE', #29291 ) ;
#5235=DIRECTION ( 'NONE',  ( -0.000000000000000000, -0.000000000000000000, 1.000000000000000000 ) ) ;
#5250=EDGE_CURVE ( 'NONE', #10573, #33855, #14011, .T. ) ;
#5252=CARTESIAN_POINT ( 'NONE',  ( 8.707710598626619003, 8.357316531739471088, 159.5815388724490163 ) ) ;
#5262=CARTESIAN_POINT ( 'NONE',  ( -10.27611701369020381, 22.27821838569869684, 159.5815388724490163 ) ) ;
#5266=DIRECTION ( 'NONE',  ( 1.000000000000000000, 0.000000000000000000, 0.000000000000000000 ) ) ;
#5272=LINE ( 'NONE', #18245, #15345 ) ;
#5347=CARTESIAN_POINT ( 'NONE',  ( -1.196959198423996895E-13, 28.72222769588706015, 159.5815388724490163 ) ) ;
#5354=ORIENTED_EDGE ( 'NONE', *, *, #37531, .F. ) ;
#5368=PLANE ( 'NONE',  #26208 ) ;
#5385=CYLINDRICAL_SURFACE ( 'NONE', #41601, 7.579174044924941178 ) ;
#5391=CARTESIAN_POINT ( 'NONE',  ( 2.437533878364066098, 4.288089548799034922, 153.3425884160446913 ) ) ;
#5400=CARTESIAN_POINT ( 'NONE',  ( 13.87973638471548199, 18.10731986427940043, 153.6269493541824431 ) ) ;
#5407=CARTESIAN_POINT ( 'NONE',  ( -5.209739300208506840, 26.52353316214900047, 164.5815388724490163 ) ) ;
#5409=VECTOR ( 'NONE', #70, 1000.000000000000000 ) ;
#5425=CARTESIAN_POINT ( 'NONE',  ( -13.06543980208727618, 21.74250979011898366, 150.5815388724490163 ) ) ;
#5451=VERTEX_POINT ( 'NONE', #41793 ) ;
#5460=CIRCLE ( 'NONE', #12228, 5.000000000000004441 ) ;
#5467=ORIENTED_EDGE ( 'NONE', *, *, #34009, .F. ) ;
#5515=B_SPLINE_CURVE_WITH_KNOTS ( 'NONE', 3,
 ( #25842, #22428, #25635, #6270, #35820, #29213, #35406, #88, #32419, #3286, #32621, #22850, #6681, #32002, #19861, #19652 ),
 .UNSPECIFIED., .F., .F.,
 ( 4, 2, 2, 2, 2, 2, 2, 4 ),
 ( 2.540748634406939408E-07, 0.001910996430635847169, 0.002866367608522052499, 0.003821738786408257395, 0.004777109964294461858, 0.005732481142180667621, 0.006687852320066871650, 0.007643223497953077414 ),
 .UNSPECIFIED. ) ;
#5552=VERTEX_POINT ( 'NONE', #930 ) ;
#5557=DIRECTION ( 'NONE',  ( -1.000000000000000000, 0.000000000000000000, -0.000000000000000000 ) ) ;
#5561=CARTESIAN_POINT ( 'NONE',  ( -2.858598646996159509, 4.063742324715557075, 150.5815388724490163 ) ) ;
#5641=CARTESIAN_POINT ( 'NONE',  ( -9.535873231784242066, 10.83976048429175520, 154.5815388724490163 ) ) ;
#5671=CIRCLE ( 'NONE', #11787, 5.000000000000000000 ) ;
#5676=AXIS2_PLACEMENT_3D ( 'NONE', #1682, #40183, #34015 ) ;
#5699=PLANE ( 'NONE',  #42098 ) ;
#5741=CARTESIAN_POINT ( 'NONE',  ( 7.887293579986041969, 6.217443341193099826, 153.5499870077387357 ) ) ;
#5757=AXIS2_PLACEMENT_3D ( 'NONE', #38059, #38265, #41469 ) ;
#5758=ORIENTED_EDGE ( 'NONE', *, *, #30153, .F. ) ;
#5764=LINE ( 'NONE', #18312, #26384 ) ;
#5778=CARTESIAN_POINT ( 'NONE',  ( 16.28249153430137852, 26.90070087040669122, 159.5815388724490163 ) ) ;
#5779=ADVANCED_FACE ( 'NONE', ( #34507 ), #4247, .T. ) ;
#5782=ORIENTED_EDGE ( 'NONE', *, *, #20269, .F. ) ;
#5785=EDGE_CURVE ( 'NONE', #40356, #29125, #37706, .T. ) ;
#5795=SPHERICAL_SURFACE ( 'NONE', #28267, 5.000000000000000000 ) ;
#5801=ORIENTED_EDGE ( 'NONE', *, *, #15562, .F. ) ;
#5807=LINE ( 'NONE', #22380, #21968 ) ;
#5813=CARTESIAN_POINT ( 'NONE',  ( 5.453575347710441612, 3.477978550085004006, 154.3405383141646610 ) ) ;
#5815=FACE_OUTER_BOUND ( 'NONE', #12151, .T. ) ;
#5846=CARTESIAN_POINT ( 'NONE',  ( 2.302507646137074410E-15, -1.301401740813418195, 159.5815388724490163 ) ) ;
#5863=DIRECTION ( 'NONE',  ( 1.000000000000000000, 0.000000000000000000, 0.000000000000000000 ) ) ;
#5868=DIRECTION ( 'NONE',  ( -0.03404294460293532526, -0.9994203709764784005, -0.000000000000000000 ) ) ;
#5883=CARTESIAN_POINT ( 'NONE',  ( -15.19729569207834885, 16.01032910557492883, 154.4794923609106263 ) ) ;
#5905=CARTESIAN_POINT ( 'NONE',  ( 10.03587323178444279, 11.70578588807654441, 154.5815388724490163 ) ) ;
#5920=CARTESIAN_POINT ( 'NONE',  ( -1.263023857913828651, 28.82150479573344981, 152.0797566321132877 ) ) ;
#5940=DIRECTION ( 'NONE',  ( -0.000000000000000000, -0.000000000000000000, -1.000000000000000000 ) ) ;
#5947=CARTESIAN_POINT ( 'NONE',  ( -3.563940842959833599, 29.61244032134267101, 152.8454421597756152 ) ) ;
#5964=EDGE_CURVE ( 'NONE', #7502, #37842, #13217, .T. ) ;
#6002=SPHERICAL_SURFACE ( 'NONE', #6280, 5.000000000000000000 ) ;
#6010=DIRECTION ( 'NONE',  ( 0.8660254037844363761, 0.5000000000000039968, 0.000000000000000000 ) ) ;
#6012=VECTOR ( 'NONE', #17948, 1000.000000000000000 ) ;
#6013=ORIENTED_EDGE ( 'NONE', *, *, #18837, .T. ) ;
#6032=CARTESIAN_POINT ( 'NONE',  ( -10.53587323178440194, 22.42818870813906429, 154.5815388724490163 ) ) ;
#6038=VECTOR ( 'NONE', #4845, 1000.000000000000000 ) ;
#6085=EDGE_LOOP ( 'NONE', ( #11414, #37575, #17555, #10379, #42068, #16911 ) ) ;
#6102=EDGE_CURVE ( 'NONE', #18422, #40121, #27351, .T. ) ;
#6105=DIRECTION ( 'NONE',  ( 1.000000000000000000, 0.000000000000000000, 0.000000000000000000 ) ) ;
#6120=CARTESIAN_POINT ( 'NONE',  ( -9.276117013690740265, 10.98973080673171765, 154.5815388724490163 ) ) ;
#6123=CARTESIAN_POINT ( 'NONE',  ( 10.27611701369066921, 12.72178161430110066, 154.5815388724490163 ) ) ;
#6126=CARTESIAN_POINT ( 'NONE',  ( -8.372639320098761218, 6.970599522130121350, 153.3561523384327927 ) ) ;
#6127=VERTEX_POINT ( 'NONE', #29366 ) ;
#6128=CARTESIAN_POINT ( 'NONE',  ( -5.970050184154961137, 29.94329617374863517, 153.5717503611250550 ) ) ;
#6129=CARTESIAN_POINT ( 'NONE',  ( 3.563940842959894884, 5.387559678655694739, 152.8454421597760700 ) ) ;
#6138=CARTESIAN_POINT ( 'NONE',  ( 13.12940535518733931, 15.28010775066634608, 153.2716026109635266 ) ) ;
#6161=DIRECTION ( 'NONE',  ( -0.000000000000000000, -0.000000000000000000, -1.000000000000000000 ) ) ;
#6187=AXIS2_PLACEMENT_3D ( 'NONE', #21139, #4969, #17951 ) ;
#6193=EDGE_CURVE ( 'NONE', #7487, #28419, #32984, .T. ) ;
#6205=CARTESIAN_POINT ( 'NONE',  ( 9.718734271691504389, 23.11111384794381252, 154.5815388724490163 ) ) ;
#6214=CARTESIAN_POINT ( 'NONE',  ( 14.54815605848642690, 14.67187636176522858, 154.2016373142949988 ) ) ;
#6236=ADVANCED_FACE ( 'NONE', ( #29793 ), #37036, .T. ) ;
#6249=CARTESIAN_POINT ( 'NONE',  ( 8.707710598625942211, 26.64268346825921085, 152.8454421597755015 ) ) ;
#6250=DIRECTION ( 'NONE',  ( 0.000000000000000000, -0.000000000000000000, -1.000000000000000000 ) ) ;
#6258=CARTESIAN_POINT ( 'NONE',  ( 2.302507646137074410E-15, -1.301401740813418195, 159.5815388724490163 ) ) ;
#6270=CARTESIAN_POINT ( 'NONE',  ( -10.64649782989250504, 13.17637234917139644, 152.1415020206854365 ) ) ;
#6280=AXIS2_PLACEMENT_3D ( 'NONE', #12802, #9408, #38752 ) ;
#6288=ORIENTED_EDGE ( 'NONE', *, *, #6779, .T. ) ;
#6293=VERTEX_POINT ( 'NONE', #23858 ) ;
#6313=CARTESIAN_POINT ( 'NONE',  ( -9.067620284531709984, 24.55832382288969029, 152.1415020426161675 ) ) ;
#6319=CARTESIAN_POINT ( 'NONE',  ( 14.66485744952540315, 20.14980920382255292, 154.2521761610834119 ) ) ;
#6320=CARTESIAN_POINT ( 'NONE',  ( -13.91947860041774376, 17.49999999999951683, 153.6452861111158086 ) ) ;
#6336=CARTESIAN_POINT ( 'NONE',  ( -7.326644855052485639, 31.07431547527046334, 154.5725613197531629 ) ) ;
#6345=AXIS2_PLACEMENT_3D ( 'NONE', #22235, #5235, #18420 ) ;
#6352=CARTESIAN_POINT ( 'NONE',  ( 13.91947860041720908, 17.49999999999956302, 153.6452861111154675 ) ) ;
#6357=CARTESIAN_POINT ( 'NONE',  ( 9.724190303529367085, 28.68314134458470832, 154.2011257354760687 ) ) ;
#6381=CARTESIAN_POINT ( 'NONE',  ( -0.2606827522253820639, 30.22248532900398033, 152.9052493585880086 ) ) ;
#6394=B_SPLINE_CURVE_WITH_KNOTS ( 'NONE', 3,
 ( #16243, #36858, #40249, #17502, #29828, #696, #24102, #4520, #33447, #39392, #913, #36640, #7504, #36204, #481, #23892 ),
 .UNSPECIFIED., .F., .F.,
 ( 4, 2, 2, 2, 2, 2, 2, 4 ),
 ( 2.508354784748761536E-07, 0.001523425935721370523, 0.002285013485842823672, 0.003046601035964277039, 0.003808188586085729972, 0.004569776136207182905, 0.005331363686328636706, 0.006092951236450089639 ),
 .UNSPECIFIED. ) ;
#6422=TOROIDAL_SURFACE ( 'NONE', #7085, 11.07917404492516233, 5.000000000000000000 ) ;
#6433=DIRECTION ( 'NONE',  ( 0.000000000000000000, 0.000000000000000000, -1.000000000000000000 ) ) ;
#6437=EDGE_CURVE ( 'NONE', #4399, #26696, #8869, .T. ) ;
#6438=DIRECTION ( 'NONE',  ( -0.000000000000000000, -0.000000000000000000, -1.000000000000000000 ) ) ;
#6513=EDGE_LOOP ( 'NONE', ( #24766, #35324, #20209 ) ) ;
#6530=DIRECTION ( 'NONE',  ( -1.000000000000000000, 0.000000000000000000, 0.000000000000000000 ) ) ;
#6532=EDGE_CURVE ( 'NONE', #6594, #2798, #25088, .T. ) ;
#6536=CARTESIAN_POINT ( 'NONE',  ( 11.75845712892196637, 12.16770857437972353, 153.0204462570416979 ) ) ;
#6544=VERTEX_POINT ( 'NONE', #28692 ) ;
#6567=CARTESIAN_POINT ( 'NONE',  ( 13.87922053742511075, 16.89024087513384487, 153.6267098343898851 ) ) ;
#6593=CARTESIAN_POINT ( 'NONE',  ( 1.974753549812969577, 30.54673820232729398, 153.1965160626530178 ) ) ;
#6594=VERTEX_POINT ( 'NONE', #3387 ) ;
#6611=ORIENTED_EDGE ( 'NONE', *, *, #27932, .F. ) ;
#6644=CARTESIAN_POINT ( 'NONE',  ( 9.957960250865429686, 6.896283818747226846, 154.0322826691240152 ) ) ;
#6656=AXIS2_PLACEMENT_3D ( 'NONE', #29537, #26359, #10189 ) ;
#6663=LINE ( 'NONE', #19225, #33246 ) ;
#6681=CARTESIAN_POINT ( 'NONE',  ( -8.836825633740376773, 9.547522263686650135, 152.3877645506826468 ) ) ;
#6682=CARTESIAN_POINT ( 'NONE',  ( 0.000000000000000000, 17.49999999999998934, 159.5815388724490163 ) ) ;
#6705=AXIS2_PLACEMENT_3D ( 'NONE', #39600, #32587, #3452 ) ;
#6710=EDGE_LOOP ( 'NONE', ( #29458, #21202, #22666, #38007, #28770, #2893, #12081, #1875, #21194, #4308, #41980, #4873, #16857, #15717, #16433, #41926 ) ) ;
#6714=ADVANCED_FACE ( 'NONE', ( #33798 ), #10619, .F. ) ;
#6730=EDGE_CURVE ( 'NONE', #38421, #37104, #10730, .T. ) ;
#6734=CARTESIAN_POINT ( 'NONE',  ( -12.51134252589945461, 20.32026673028943975, 152.9677466506648784 ) ) ;
#6736=CARTESIAN_POINT ( 'NONE',  ( -5.209739300208506840, 26.52353316214900047, 159.5815388724490163 ) ) ;
#6764=ADVANCED_FACE ( 'NONE', ( #6997 ), #23382, .T. ) ;
#6772=VECTOR ( 'NONE', #39592, 1000.000000000000000 ) ;
#6779=EDGE_CURVE ( 'NONE', #29296, #2682, #12788, .T. ) ;
#6795=CARTESIAN_POINT ( 'NONE',  ( -1.012168522246219782, 30.30180045204023287, 152.9774433921726882 ) ) ;
#6811=ORIENTED_EDGE ( 'NONE', *, *, #11547, .F. ) ;
#6828=CIRCLE ( 'NONE', #11600, 5.000000000000000000 ) ;
#6831=CARTESIAN_POINT ( 'NONE',  ( 8.707710598626619003, 8.357316531739469312, 152.8454421597759847 ) ) ;
#6849=CARTESIAN_POINT ( 'NONE',  ( 9.292375245848642606, 5.582027987049082540, 154.3820435809093397 ) ) ;
#6864=DIRECTION ( 'NONE',  ( 0.000000000000000000, 0.000000000000000000, -1.000000000000000000 ) ) ;
#6896=EDGE_CURVE ( 'NONE', #5451, #17600, #35196, .T. ) ;
#6911=ORIENTED_EDGE ( 'NONE', *, *, #685, .T. ) ;
#6935=CARTESIAN_POINT ( 'NONE',  ( 0.000000000000000000, 17.49999999999998934, 159.5815388724490163 ) ) ;
#6937=FACE_OUTER_BOUND ( 'NONE', #14668, .T. ) ;
#6944=CARTESIAN_POINT ( 'NONE',  ( 13.40983285079566478, 21.52771932643388197, 153.6939610446745519 ) ) ;
#6945=CARTESIAN_POINT ( 'NONE',  ( -13.76218140321603656, 18.54844794216283077, 153.5721917427166829 ) ) ;
#6952=DIRECTION ( 'NONE',  ( -0.000000000000000000, -0.000000000000000000, 1.000000000000000000 ) ) ;
#6962=CARTESIAN_POINT ( 'NONE',  ( -9.411389837926479984, 29.24216370071915705, 154.3424624685361266 ) ) ;
#6976=CARTESIAN_POINT ( 'NONE',  ( 0.000000000000000000, 34.99999999999997868, 154.5815388724490163 ) ) ;
#6980=CIRCLE ( 'NONE', #15788, 7.579174044925158782 ) ;
#6997=FACE_OUTER_BOUND ( 'NONE', #7456, .T. ) ;
#7005=AXIS2_PLACEMENT_3D ( 'NONE', #8058, #36564, #33368 ) ;
#7008=B_SPLINE_CURVE_WITH_KNOTS ( 'NONE', 3,
 ( #32843, #17331, #19665, #13922, #39434, #14134, #27109, #13711, #23282, #3923, #10105, #16698, #20093, #36678 ),
 .UNSPECIFIED., .F., .F.,
 ( 4, 2, 2, 2, 2, 2, 4 ),
 ( 0.003646029068602594809, 0.004555261728908261559, 0.005009878059061094284, 0.005464494389213927876, 0.005919110719366760601, 0.006373727049519594193, 0.007282959709825263979 ),
 .UNSPECIFIED. ) ;
#7011=CARTESIAN_POINT ( 'NONE',  ( 1.254681948488747034, 30.34790559804115873, 153.0192156368753444 ) ) ;
#7038=FACE_OUTER_BOUND ( 'NONE', #34172, .T. ) ;
#7085=AXIS2_PLACEMENT_3D ( 'NONE', #14647, #7848, #5266 ) ;
#7106=DIRECTION ( 'NONE',  ( -1.000000000000000000, 0.000000000000000000, 0.000000000000000000 ) ) ;
#7113=LINE ( 'NONE', #20295, #12992 ) ;
#7128=ORIENTED_EDGE ( 'NONE', *, *, #32380, .T. ) ;
#7135=AXIS2_PLACEMENT_3D ( 'NONE', #8658, #11636, #15268 ) ;
#7163=CARTESIAN_POINT ( 'NONE',  ( 12.28238916904378719, 12.70424003126727541, 153.1863241608643875 ) ) ;
#7164=CARTESIAN_POINT ( 'NONE',  ( -12.73238323000468597, 20.14266894880929115, 153.0776982460621127 ) ) ;
#7166=CYLINDRICAL_SURFACE ( 'NONE', #21429, 3.500000000000001332 ) ;
#7192=EDGE_LOOP ( 'NONE', ( #34117, #24725, #15931, #11677 ) ) ;
#7212=FACE_OUTER_BOUND ( 'NONE', #25185, .T. ) ;
#7229=DIRECTION ( 'NONE',  ( 1.000000000000000000, 0.000000000000000000, 0.000000000000000000 ) ) ;
#7234=AXIS2_PLACEMENT_3D ( 'NONE', #6976, #38675, #35898 ) ;
#7255=DIRECTION ( 'NONE',  ( -0.000000000000000000, 0.000000000000000000, -1.000000000000000000 ) ) ;
#7278=CARTESIAN_POINT ( 'NONE',  ( 5.977173621345689192, 29.94174207387652942, 153.5727845806729022 ) ) ;
#7286=CARTESIAN_POINT ( 'NONE',  ( 11.75395375419299171, 22.83736619992661332, 153.0192156799700172 ) ) ;
#7290=ORIENTED_EDGE ( 'NONE', *, *, #10006, .F. ) ;
#7318=FACE_OUTER_BOUND ( 'NONE', #24148, .T. ) ;
#7394=FACE_OUTER_BOUND ( 'NONE', #22228, .T. ) ;
#7431=DIRECTION ( 'NONE',  ( -1.000000000000000000, 0.000000000000000000, 0.000000000000000000 ) ) ;
#7442=ORIENTED_EDGE ( 'NONE', *, *, #21571, .T. ) ;
#7443=CARTESIAN_POINT ( 'NONE',  ( -2.858598646996059145, 30.93625767528277848, 153.5324451153149710 ) ) ;
#7452=VERTEX_POINT ( 'NONE', #33204 ) ;
#7456=EDGE_LOOP ( 'NONE', ( #4197, #19354, #7806, #24711, #4340, #33162, #11667, #3702 ) ) ;
#7487=VERTEX_POINT ( 'NONE', #4557 ) ;
#7488=CARTESIAN_POINT ( 'NONE',  ( 9.563059451444853920, 23.38002828119538634, 151.9771748954509292 ) ) ;
#7489=CARTESIAN_POINT ( 'NONE',  ( 9.535873231784194104, 24.16023951570828032, 159.5815388724490163 ) ) ;
#7502=VERTEX_POINT ( 'NONE', #25803 ) ;
#7504=CARTESIAN_POINT ( 'NONE',  ( -10.31142999045227704, 25.73355560301168410, 153.1965159924007196 ) ) ;
#7508=DIRECTION ( 'NONE',  ( 0.000000000000000000, 0.000000000000000000, 1.000000000000000000 ) ) ;
#7526=CARTESIAN_POINT ( 'NONE',  ( -8.707710598626182019, 26.64268346825927836, 152.8454421597756436 ) ) ;
#7532=DIRECTION ( 'NONE',  ( 0.5000000000000101030, -0.8660254037844328234, 0.000000000000000000 ) ) ;
#7544=ORIENTED_EDGE ( 'NONE', *, *, #26480, .T. ) ;
#7563=PLANE ( 'NONE',  #36725 ) ;
#7609=CIRCLE ( 'NONE', #13037, 5.000000000000004441 ) ;
#7620=AXIS2_PLACEMENT_3D ( 'NONE', #10838, #4244, #11454 ) ;
#7628=CARTESIAN_POINT ( 'NONE',  ( -4.330127018922124371, 14.99999999999985789, 154.5815388724490163 ) ) ;
#7643=CARTESIAN_POINT ( 'NONE',  ( 10.41947860041720908, 17.49999999999956302, 159.5815388724490163 ) ) ;
#7656=CARTESIAN_POINT ( 'NONE',  ( 0.000000000000000000, 17.49999999999998934, 159.5815388724490163 ) ) ;
#7665=PLANE ( 'NONE',  #26020 ) ;
#7702=LINE ( 'NONE', #7489, #6772 ) ;
#7716=AXIS2_PLACEMENT_3D ( 'NONE', #12512, #9105, #38458 ) ;
#7721=AXIS2_PLACEMENT_3D ( 'NONE', #35970, #36401, #29590 ) ;
#7740=CARTESIAN_POINT ( 'NONE',  ( 13.72762536464759187, 13.72808788916961475, 153.8384576237820909 ) ) ;
#7742=ADVANCED_FACE ( 'NONE', ( #15339 ), #5795, .T. ) ;
#7752=DIRECTION ( 'NONE',  ( -0.000000000000000000, -0.000000000000000000, -1.000000000000000000 ) ) ;
#7760=CARTESIAN_POINT ( 'NONE',  ( -0.2485248900957898466, 4.778023858538846369, 152.9047840822885576 ) ) ;
#7767=ORIENTED_EDGE ( 'NONE', *, *, #41629, .T. ) ;
#7793=EDGE_CURVE ( 'NONE', #8962, #6293, #14372, .T. ) ;
#7806=ORIENTED_EDGE ( 'NONE', *, *, #10006, .T. ) ;
#7821=CIRCLE ( 'NONE', #30242, 5.000000000000004441 ) ;
#7848=DIRECTION ( 'NONE',  ( -0.000000000000000000, 0.000000000000000000, 1.000000000000000000 ) ) ;
#7863=DIRECTION ( 'NONE',  ( 0.000000000000000000, 0.000000000000000000, 1.000000000000000000 ) ) ;
#7869=DIRECTION ( 'NONE',  ( -0.000000000000000000, -0.000000000000000000, -1.000000000000000000 ) ) ;
#7891=CARTESIAN_POINT ( 'NONE',  ( 2.302507646137074410E-15, -1.301401740813418195, 159.5815388724490163 ) ) ;
#7892=DIRECTION ( 'NONE',  ( 0.8660254037844397068, -0.4999999999999979461, 0.000000000000000000 ) ) ;
#7910=DIRECTION ( 'NONE',  ( -0.000000000000000000, -0.000000000000000000, 1.000000000000000000 ) ) ;
#7916=ORIENTED_EDGE ( 'NONE', *, *, #19738, .F. ) ;
#7918=CARTESIAN_POINT ( 'NONE',  ( 8.372639320097622573, 28.02940047786812983, 153.3561523384319401 ) ) ;
#7923=ADVANCED_FACE ( 'NONE', ( #26168 ), #19769, .F. ) ;
#7940=ADVANCED_FACE ( 'NONE', ( #14666 ), #30189, .F. ) ;
#7990=LINE ( 'NONE', #20962, #4839 ) ;
#7991=EDGE_CURVE ( 'NONE', #4671, #12772, #24036, .T. ) ;
#8024=EDGE_LOOP ( 'NONE', ( #1741, #16609, #15313, #20041 ) ) ;
#8048=CARTESIAN_POINT ( 'NONE',  ( -3.742640687119191512, 14.18448485343225585, 154.5815388724490163 ) ) ;
#8058=CARTESIAN_POINT ( 'NONE',  ( 0.000000000000000000, 17.49999999999998934, 159.5815388724490163 ) ) ;
#8059=SPHERICAL_SURFACE ( 'NONE', #26060, 5.000000000000000000 ) ;
#8071=ORIENTED_EDGE ( 'NONE', *, *, #32906, .F. ) ;
#8074=CARTESIAN_POINT ( 'NONE',  ( 2.302507646137074410E-15, -1.301401740813418195, 164.5815388724490163 ) ) ;
#8092=DIRECTION ( 'NONE',  ( 0.000000000000000000, -0.000000000000000000, -1.000000000000000000 ) ) ;
#8109=AXIS2_PLACEMENT_3D ( 'NONE', #41484, #22751, #38278 ) ;
#8117=VERTEX_POINT ( 'NONE', #6123 ) ;
#8163=SPHERICAL_SURFACE ( 'NONE', #6187, 5.000000000000000000 ) ;
#8166=CARTESIAN_POINT ( 'NONE',  ( -2.647879461657173916, 4.176015466079334715, 153.4374325377220885 ) ) ;
#8168=VERTEX_POINT ( 'NONE', #34426 ) ;
#8177=EDGE_CURVE ( 'NONE', #13562, #28722, #16559, .T. ) ;
#8183=CARTESIAN_POINT ( 'NONE',  ( -9.718734271692440529, 11.88888615205571320, 154.5815388724490163 ) ) ;
#8228=AXIS2_PLACEMENT_3D ( 'NONE', #40168, #24429, #27411 ) ;
#8278=VERTEX_POINT ( 'NONE', #2515 ) ;
#8288=AXIS2_PLACEMENT_3D ( 'NONE', #39020, #32227, #3095 ) ;
#8334=AXIS2_PLACEMENT_3D ( 'NONE', #23203, #20443, #14486 ) ;
#8364=CARTESIAN_POINT ( 'NONE',  ( 16.28249153430138207, 8.099299129593287461, 159.5815388724490163 ) ) ;
#8366=CARTESIAN_POINT ( 'NONE',  ( 9.030446397028940808, 5.244147267330249385, 154.4507089031957889 ) ) ;
#8369=AXIS2_PLACEMENT_3D ( 'NONE', #35452, #22689, #23102 ) ;
#8380=ORIENTED_EDGE ( 'NONE', *, *, #23895, .F. ) ;
#8399=VECTOR ( 'NONE', #10882, 1000.000000000000000 ) ;
#8421=ORIENTED_EDGE ( 'NONE', *, *, #39884, .T. ) ;
#8446=EDGE_CURVE ( 'NONE', #8962, #19866, #13391, .T. ) ;
#8464=ORIENTED_EDGE ( 'NONE', *, *, #40413, .F. ) ;
#8478=CARTESIAN_POINT ( 'NONE',  ( -13.06543980208727262, 21.74250979011898721, 153.5324451153151983 ) ) ;
#8517=CARTESIAN_POINT ( 'NONE',  ( 10.41947860041720730, 17.49999999999956302, 164.5815388724490163 ) ) ;
#8520=CARTESIAN_POINT ( 'NONE',  ( -3.563940842960075184, 5.387559678655594375, 152.8454421597761552 ) ) ;
#8540=LINE ( 'NONE', #5561, #31445 ) ;
#8546=CARTESIAN_POINT ( 'NONE',  ( -3.742640687119191512, 14.18448485343225585, 155.5815388724490163 ) ) ;
#8562=ADVANCED_FACE ( 'NONE', ( #4612 ), #34163, .T. ) ;
#8586=CIRCLE ( 'NONE', #1129, 5.000000000000000888 ) ;
#8628=DIRECTION ( 'NONE',  ( -0.000000000000000000, 0.000000000000000000, 1.000000000000000000 ) ) ;
#8642=ORIENTED_EDGE ( 'NONE', *, *, #26666, .T. ) ;
#8658=CARTESIAN_POINT ( 'NONE',  ( -5.209739300209234258, 8.476466837849004676, 159.5815388724490163 ) ) ;
#8682=CARTESIAN_POINT ( 'NONE',  ( 3.042470621311043288, 29.33459613825148438, 152.5896212286789364 ) ) ;
#8691=EDGE_CURVE ( 'NONE', #27377, #36248, #27983, .T. ) ;
#8699=VERTEX_POINT ( 'NONE', #2670 ) ;
#8712=CARTESIAN_POINT ( 'NONE',  ( 5.373768961465674288, 4.977207596738975504, 153.4640811590195426 ) ) ;
#8726=DIRECTION ( 'NONE',  ( 1.000000000000000000, 0.000000000000000000, 0.000000000000000000 ) ) ;
#8733=DIRECTION ( 'NONE',  ( 1.000000000000000000, 0.000000000000000000, 0.000000000000000000 ) ) ;
#8738=CARTESIAN_POINT ( 'NONE',  ( -8.707710598626928089, 8.357316531739311216, 159.5815388724490163 ) ) ;
#8752=ORIENTED_EDGE ( 'NONE', *, *, #18414, .T. ) ;
#8765=B_SPLINE_CURVE_WITH_KNOTS ( 'NONE', 3,
 ( #29268, #6734, #7164, #13755, #39063, #140, #38859, #39694, #39479, #35459, #6945, #25894, #3751, #6320 ),
 .UNSPECIFIED., .F., .F.,
 ( 4, 2, 2, 2, 2, 2, 4 ),
 ( 2.534995934260133079E-07, 0.0009116973918457152134, 0.001367419337971863312, 0.001823141284098011737, 0.002278863230224159944, 0.002734585176350307935, 0.003646029068602594809 ),
 .UNSPECIFIED. ) ;
#8794=PLANE ( 'NONE',  #28590 ) ;
#8798=ORIENTED_EDGE ( 'NONE', *, *, #4636, .F. ) ;
#8803=ORIENTED_EDGE ( 'NONE', *, *, #33688, .T. ) ;
#8811=ORIENTED_EDGE ( 'NONE', *, *, #32189, .F. ) ;
#8844=PRODUCT_DEFINITION ( 'UNKNOWN', '', #36370, #16523 ) ;
#8860=CARTESIAN_POINT ( 'NONE',  ( -14.66485744952595738, 14.85019079617655180, 154.2521761610838666 ) ) ;
#8869=B_SPLINE_CURVE_WITH_KNOTS ( 'NONE', 3,
 ( #15106, #25100, #21686, #18287, #28069, #21481, #31058, #8712, #15324, #41262, #34453, #41049, #11901, #24894, #11483, #38064, #5741, #8922, #14696, #2337, #27860, #40836, #1910, #18086, #11688, #34660 ),
 .UNSPECIFIED., .F., .F.,
 ( 4, 2, 2, 2, 2, 2, 2, 2, 2, 2, 2, 2, 4 ),
 ( 2.437304301980259244E-07, 0.0009105819918573546459, 0.001365751122570934423, 0.001820920253284514199, 0.002276089383998093976, 0.002731258514711673753, 0.003641596776138843281, 0.004551935037566012809, 0.005007104168279592586, 0.005462273298993172363, 0.005917442429706752140, 0.006372611560420331916, 0.007282949821847491470 ),
 .UNSPECIFIED. ) ;
#8883=ORIENTED_EDGE ( 'NONE', *, *, #23219, .T. ) ;
#8903=ORIENTED_EDGE ( 'NONE', *, *, #8446, .F. ) ;
#8907=DIRECTION ( 'NONE',  ( -1.000000000000000000, 0.000000000000000000, 0.000000000000000000 ) ) ;
#8922=CARTESIAN_POINT ( 'NONE',  ( 8.070690082936398113, 6.454723852599054013, 153.4965620064461120 ) ) ;
#8937=ORIENTED_EDGE ( 'NONE', *, *, #5140, .F. ) ;
#8938=FACE_OUTER_BOUND ( 'NONE', #8024, .T. ) ;
#8946=DIRECTION ( 'NONE',  ( -0.000000000000000000, -0.000000000000000000, -1.000000000000000000 ) ) ;
#8962=VERTEX_POINT ( 'NONE', #7443 ) ;
#8982=CARTESIAN_POINT ( 'NONE',  ( 14.29598812252905482, 14.33504584695328532, 154.0913471354969317 ) ) ;
#8985=LINE ( 'NONE', #21958, #23411 ) ;
#9007=VERTEX_POINT ( 'NONE', #26175 ) ;
#9009=CARTESIAN_POINT ( 'NONE',  ( 13.59976475949342678, 18.96908283097675962, 153.4960580910866668 ) ) ;
#9013=FACE_OUTER_BOUND ( 'NONE', #28937, .T. ) ;
#9018=EDGE_CURVE ( 'NONE', #29125, #18650, #224, .T. ) ;
#9069=ORIENTED_EDGE ( 'NONE', *, *, #6779, .F. ) ;
#9081=CARTESIAN_POINT ( 'NONE',  ( -15.41947860041774376, 17.49999999999951683, 150.5815388724490163 ) ) ;
#9096=EDGE_LOOP ( 'NONE', ( #7544, #4616 ) ) ;
#9102=DIRECTION ( 'NONE',  ( -0.000000000000000000, -0.000000000000000000, -1.000000000000000000 ) ) ;
#9105=DIRECTION ( 'NONE',  ( 0.000000000000000000, -0.000000000000000000, -1.000000000000000000 ) ) ;
#9118=VECTOR ( 'NONE', #22891, 1000.000000000000000 ) ;
#9150=VERTEX_POINT ( 'NONE', #23830 ) ;
#9160=VERTEX_POINT ( 'NONE', #8478 ) ;
#9163=AXIS2_PLACEMENT_3D ( 'NONE', #21430, #2068, #31829 ) ;
#9177=VERTEX_POINT ( 'NONE', #4874 ) ;
#9195=ORIENTED_EDGE ( 'NONE', *, *, #6102, .F. ) ;
#9208=EDGE_CURVE ( 'NONE', #35160, #19636, #2880, .T. ) ;
#9229=ADVANCED_FACE ( 'NONE', ( #38671 ), #27356, .T. ) ;
#9232=EDGE_CURVE ( 'NONE', #13300, #26392, #34813, .T. ) ;
#9261=AXIS2_PLACEMENT_3D ( 'NONE', #27595, #30149, #17607 ) ;
#9301=CYLINDRICAL_SURFACE ( 'NONE', #1007, 6.079174044926337395 ) ;
#9324=EDGE_CURVE ( 'NONE', #645, #4399, #38693, .T. ) ;
#9328=CARTESIAN_POINT ( 'NONE',  ( -6.408084924487074119, 29.82586181747419118, 153.6264000693442711 ) ) ;
#9329=CARTESIAN_POINT ( 'NONE',  ( 3.032103446743008579, 5.651413488468350010, 152.5993403105697723 ) ) ;
#9341=ORIENTED_EDGE ( 'NONE', *, *, #31880, .T. ) ;
#9364=EDGE_LOOP ( 'NONE', ( #2468, #1575, #39871, #29144 ) ) ;
#9374=ORIENTED_EDGE ( 'NONE', *, *, #17306, .F. ) ;
#9408=DIRECTION ( 'NONE',  ( 0.000000000000000000, 1.000000000000000000, 0.000000000000000000 ) ) ;
#9409=EDGE_LOOP ( 'NONE', ( #34333, #13294, #17956, #15810 ) ) ;
#9440=VECTOR ( 'NONE', #38897, 1000.000000000000000 ) ;
#9441=CARTESIAN_POINT ( 'NONE',  ( -16.28249153430137497, 8.099299129593275026, 164.5815388724490163 ) ) ;
#9449=DIRECTION ( 'NONE',  ( -0.000000000000000000, 0.000000000000000000, 1.000000000000000000 ) ) ;
#9468=ORIENTED_EDGE ( 'NONE', *, *, #30153, .T. ) ;
#9480=EDGE_LOOP ( 'NONE', ( #38193, #2998, #26283, #21255, #1323, #1633 ) ) ;
#9509=PLANE ( 'NONE',  #8369 ) ;
#9511=DIRECTION ( 'NONE',  ( 1.000000000000000000, 0.000000000000000000, 0.000000000000000000 ) ) ;
#9518=FACE_OUTER_BOUND ( 'NONE', #12461, .T. ) ;
#9531=FACE_OUTER_BOUND ( 'NONE', #15866, .T. ) ;
#9540=CARTESIAN_POINT ( 'NONE',  ( -6.697448051448398054, 5.293492502434390623, 153.6454670853914877 ) ) ;
#9567=AXIS2_PLACEMENT_3D ( 'NONE', #24751, #15392, #15170 ) ;
#9598=AXIS2_PLACEMENT_3D ( 'NONE', #1738, #30665, #8733 ) ;
#9620=DIRECTION ( 'NONE',  ( 1.000000000000000000, 0.000000000000000000, 0.000000000000000000 ) ) ;
#9626=ADVANCED_FACE ( 'NONE', ( #7394 ), #30566, .T. ) ;
#9656=LINE ( 'NONE', #35382, #5070 ) ;
#9689=VECTOR ( 'NONE', #38746, 1000.000000000000000 ) ;
#9723=CARTESIAN_POINT ( 'NONE',  ( 15.97057991159785217, 17.49999999999956302, 154.9135024962512546 ) ) ;
#9729=CARTESIAN_POINT ( 'NONE',  ( -11.77722871187752141, 20.79841459146082272, 152.5993403437912264 ) ) ;
#9735=CARTESIAN_POINT ( 'NONE',  ( 14.54810494377324481, 20.32819496402379045, 154.2016150273000221 ) ) ;
#9736=DIRECTION ( 'NONE',  ( -0.000000000000000000, -0.000000000000000000, -1.000000000000000000 ) ) ;
#9751=CARTESIAN_POINT ( 'NONE',  ( -9.626159306788924397, 28.87726500155387299, 154.2527048017821301 ) ) ;
#9755=CARTESIAN_POINT ( 'NONE',  ( -3.813105931423857342, 5.254802202609886841, 152.9676766465817934 ) ) ;
#9757=ORIENTED_EDGE ( 'NONE', *, *, #9018, .F. ) ;
#9759=AXIS2_PLACEMENT_3D ( 'NONE', #30703, #4334, #33253 ) ;
#9762=AXIS2_PLACEMENT_3D ( 'NONE', #16959, #17176, #30136 ) ;
#9763=ORIENTED_EDGE ( 'NONE', *, *, #15991, .F. ) ;
#9765=PLANE ( 'NONE',  #7234 ) ;
#9776=CARTESIAN_POINT ( 'NONE',  ( 10.13050606591841607, 27.50172420044922106, 153.8381732780032110 ) ) ;
#9786=CARTESIAN_POINT ( 'NONE',  ( 0.000000000000000000, 17.49999999999998934, 154.5815388724490163 ) ) ;
#9806=CARTESIAN_POINT ( 'NONE',  ( -13.91947860041774376, 17.49999999999951683, 159.5815388724490163 ) ) ;
#9810=DIRECTION ( 'NONE',  ( -0.000000000000000000, -0.000000000000000000, -1.000000000000000000 ) ) ;
#9816=VERTEX_POINT ( 'NONE', #1772 ) ;
#9836=VECTOR ( 'NONE', #39975, 1000.000000000000000 ) ;
#9865=CYLINDRICAL_SURFACE ( 'NONE', #38748, 7.579174044925959919 ) ;
#9870=LINE ( 'NONE', #6032, #30618 ) ;
#9918=LINE ( 'NONE', #13302, #16490 ) ;
#9934=DIRECTION ( 'NONE',  ( 1.000000000000000000, 0.000000000000000000, 0.000000000000000000 ) ) ;
#9946=CARTESIAN_POINT ( 'NONE',  ( 10.77809958360015941, 10.69197809562609791, 152.9195735126126010 ) ) ;
#9957=FACE_OUTER_BOUND ( 'NONE', #11940, .T. ) ;
#9973=CARTESIAN_POINT ( 'NONE',  ( 13.30606428308370681, 15.51524618365521491, 153.3566391844701968 ) ) ;
#9976=EDGE_CURVE ( 'NONE', #31801, #10531, #20925, .T. ) ;
#10004=CARTESIAN_POINT ( 'NONE',  ( 5.209739300208273249, 26.52353316214887968, 159.5815388724490163 ) ) ;
#10006=EDGE_CURVE ( 'NONE', #20375, #37916, #6980, .T. ) ;
#10007=ORIENTED_EDGE ( 'NONE', *, *, #16166, .T. ) ;
#10021=ORIENTED_EDGE ( 'NONE', *, *, #9208, .T. ) ;
#10047=LINE ( 'NONE', #1319, #3653 ) ;
#10059=ADVANCED_FACE ( 'NONE', ( #18559 ), #6002, .T. ) ;
#10105=CARTESIAN_POINT ( 'NONE',  ( -13.03525533431007588, 15.17011036820110981, 153.2259575457069616 ) ) ;
#10113=ORIENTED_EDGE ( 'NONE', *, *, #37103, .F. ) ;
#10133=DIRECTION ( 'NONE',  ( 0.000000000000000000, 0.000000000000000000, -1.000000000000000000 ) ) ;
#10141=LINE ( 'NONE', #10353, #36313 ) ;
#10181=CARTESIAN_POINT ( 'NONE',  ( 9.298205070445279219, 29.40977417358551094, 154.3802602823905659 ) ) ;
#10189=DIRECTION ( 'NONE',  ( -1.000000000000000000, 0.000000000000000000, 0.000000000000000000 ) ) ;
#10203=ADVANCED_BREP_SHAPE_REPRESENTATION ( '', ( #36847, #40442 ), #38405 ) ;
#10204=CARTESIAN_POINT ( 'NONE',  ( 2.647879461656943434, 30.82398453391898485, 153.4374325377216621 ) ) ;
#10212=ORIENTED_EDGE ( 'NONE', *, *, #6730, .T. ) ;
#10230=CARTESIAN_POINT ( 'NONE',  ( -1.000000000000119460, 22.39897948556632201, 159.5815388724490163 ) ) ;
#10235=CIRCLE ( 'NONE', #21114, 11.07917404492633828 ) ;
#10261=EDGE_CURVE ( 'NONE', #13719, #19636, #29371, .T. ) ;
#10275=LINE ( 'NONE', #13258, #38024 ) ;
#10319=EDGE_CURVE ( 'NONE', #26696, #11650, #25522, .T. ) ;
#10353=CARTESIAN_POINT ( 'NONE',  ( 1.196959198423996895E-13, 12.49999999999998401, 155.5815388724490163 ) ) ;
#10355=DIRECTION ( 'NONE',  ( -1.000000000000000000, 0.000000000000000000, 0.000000000000000000 ) ) ;
#10360=ORIENTED_EDGE ( 'NONE', *, *, #28217, .T. ) ;
#10379=ORIENTED_EDGE ( 'NONE', *, *, #23944, .T. ) ;
#10396=CARTESIAN_POINT ( 'NONE',  ( 5.039920647268460563, 31.52513099133343033, 154.2527047512469380 ) ) ;
#10461=CARTESIAN_POINT ( 'NONE',  ( -4.408685582965315319, 3.536562997622931803, 154.0918074332477374 ) ) ;
#10466=CARTESIAN_POINT ( 'NONE',  ( 6.417378831301363107, 29.82262957917540191, 153.6272566164921614 ) ) ;
#10467=AXIS2_PLACEMENT_3D ( 'NONE', #37666, #1929, #11501 ) ;
#10480=LINE ( 'NONE', #27071, #40289 ) ;
#10531=VERTEX_POINT ( 'NONE', #22529 ) ;
#10538=VECTOR ( 'NONE', #34820, 1000.000000000000000 ) ;
#10556=AXIS2_PLACEMENT_3D ( 'NONE', #34343, #14784, #37743 ) ;
#10561=DIRECTION ( 'NONE',  ( 1.000000000000000000, 0.000000000000000000, 0.000000000000000000 ) ) ;
#10567=LINE ( 'NONE', #29699, #24097 ) ;
#10573=VERTEX_POINT ( 'NONE', #5947 ) ;
#10599=EDGE_CURVE ( 'NONE', #37941, #9007, #18290, .T. ) ;
#10617=DIRECTION ( 'NONE',  ( -0.8485019580238489789, -0.5291922403339777148, 0.000000000000000000 ) ) ;
#10619=CYLINDRICAL_SURFACE ( 'NONE', #24345, 3.500000000000001332 ) ;
#10622=ORIENTED_EDGE ( 'NONE', *, *, #37881, .T. ) ;
#10637=EDGE_LOOP ( 'NONE', ( #640, #40758, #30457, #2042, #18121, #2098, #33182, #17805 ) ) ;
#10675=CARTESIAN_POINT ( 'NONE',  ( -8.892120608939249493, 5.087317773340616966, 154.4788437280937501 ) ) ;
#10679=CARTESIAN_POINT ( 'NONE',  ( 9.418615391892931399, 23.67094981841350076, 151.9983627776726109 ) ) ;
#10680=FACE_OUTER_BOUND ( 'NONE', #31045, .T. ) ;
#10687=ORIENTED_EDGE ( 'NONE', *, *, #8446, .T. ) ;
#10688=CARTESIAN_POINT ( 'NONE',  ( 11.59049936059900432, 23.02700438487111967, 152.9768715818104852 ) ) ;
#10692=ORIENTED_EDGE ( 'NONE', *, *, #41629, .F. ) ;
#10730=CIRCLE ( 'NONE', #6656, 7.579174044925959919 ) ;
#10736=VERTEX_POINT ( 'NONE', #19977 ) ;
#10785=PLANE ( 'NONE',  #33954 ) ;
#10794=ORIENTED_EDGE ( 'NONE', *, *, #15211, .F. ) ;
#10814=DIRECTION ( 'NONE',  ( -0.000000000000000000, -0.000000000000000000, -1.000000000000000000 ) ) ;
#10832=CARTESIAN_POINT ( 'NONE',  ( -2.858598646996055592, 30.93625767528277848, 159.5815388724490163 ) ) ;
#10838=CARTESIAN_POINT ( 'NONE',  ( -1.196959198423996895E-13, 29.08842822384727356, 154.5815388724490163 ) ) ;
#10845=VERTEX_POINT ( 'NONE', #24233 ) ;
#10852=CIRCLE ( 'NONE', #34622, 3.500000000000000000 ) ;
#10854=EDGE_CURVE ( 'NONE', #7487, #21748, #40286, .T. ) ;
#10875=ADVANCED_FACE ( 'NONE', ( #31024 ), #23603, .T. ) ;
#10882=DIRECTION ( 'NONE',  ( 0.000000000000000000, 0.000000000000000000, 1.000000000000000000 ) ) ;
#10886=CARTESIAN_POINT ( 'NONE',  ( -10.20684115509165224, 8.306252114835194433, 153.5324451153154826 ) ) ;
#10909=EDGE_CURVE ( 'NONE', #15172, #27989, #13103, .T. ) ;
#10915=CIRCLE ( 'NONE', #27907, 3.500000000000003997 ) ;
#10944=CARTESIAN_POINT ( 'NONE',  ( 1.987944452395359551, 4.465259026464273084, 153.1863241160605185 ) ) ;
#10953=EDGE_CURVE ( 'NONE', #4671, #20375, #36781, .T. ) ;
#11000=FACE_OUTER_BOUND ( 'NONE', #13648, .T. ) ;
#11017=CARTESIAN_POINT ( 'NONE',  ( -14.29598812252939055, 20.66495415304603966, 154.0913471354970739 ) ) ;
#11028=CARTESIAN_POINT ( 'NONE',  ( 10.03587323178420476, 23.29421411192385349, 154.5815388724490163 ) ) ;
#11031=CARTESIAN_POINT ( 'NONE',  ( 0.000000000000000000, 17.49999999999998934, 155.5815388724490163 ) ) ;
#11035=DIRECTION ( 'NONE',  ( 1.000000000000000000, 0.000000000000000000, 0.000000000000000000 ) ) ;
#11098=CARTESIAN_POINT ( 'NONE',  ( -5.675078561236224672, 3.493580934520590819, 154.3820435211250981 ) ) ;
#11100=PLANE ( 'NONE',  #35601 ) ;
#11104=DIRECTION ( 'NONE',  ( 0.000000000000000000, 1.000000000000000000, 0.000000000000000000 ) ) ;
#11109=CARTESIAN_POINT ( 'NONE',  ( 7.791185372433139911, 28.89186335501236869, 153.5717503904276384 ) ) ;
#11131=CARTESIAN_POINT ( 'NONE',  ( 0.000000000000000000, 0.000000000000000000, 0.000000000000000000 ) ) ;
#11149=PLANE ( 'NONE',  #19696 ) ;
#11222=ORIENTED_EDGE ( 'NONE', *, *, #18402, .F. ) ;
#11296=EDGE_CURVE ( 'NONE', #1623, #17339, #24001, .T. ) ;
#11324=VERTEX_POINT ( 'NONE', #13115 ) ;
#11327=( LENGTH_UNIT ( ) NAMED_UNIT ( * ) SI_UNIT ( .MILLI., .METRE. ) );
#11337=DIRECTION ( 'NONE',  ( 1.000000000000000000, 0.000000000000000000, 0.000000000000000000 ) ) ;
#11348=EDGE_CURVE ( 'NONE', #7502, #35681, #35862, .T. ) ;
#11349=ORIENTED_EDGE ( 'NONE', *, *, #40413, .T. ) ;
#11366=ORIENTED_EDGE ( 'NONE', *, *, #21747, .F. ) ;
#11377=EDGE_CURVE ( 'NONE', #33855, #37682, #19123, .T. ) ;
#11394=DIRECTION ( 'NONE',  ( -0.000000000000000000, -0.000000000000000000, -1.000000000000000000 ) ) ;
#11414=ORIENTED_EDGE ( 'NONE', *, *, #38040, .F. ) ;
#11421=CARTESIAN_POINT ( 'NONE',  ( 8.707710598626619003, 8.357316531739471088, 159.5815388724490163 ) ) ;
#11434=ADVANCED_FACE ( 'NONE', ( #38641 ), #9509, .F. ) ;
#11440=DIRECTION ( 'NONE',  ( -0.8505458157821428333, 1.041618210825775532E-16, 0.5259009557468868890 ) ) ;
#11442=VECTOR ( 'NONE', #4966, 1000.000000000000000 ) ;
#11454=DIRECTION ( 'NONE',  ( -0.000000000000000000, 0.000000000000000000, 1.000000000000000000 ) ) ;
#11465=CARTESIAN_POINT ( 'NONE',  ( -10.41947860041774199, 17.49999999999951683, 159.5815388724490163 ) ) ;
#11471=ORIENTED_EDGE ( 'NONE', *, *, #3835, .F. ) ;
#11483=CARTESIAN_POINT ( 'NONE',  ( 7.463020515686652701, 5.781071816537299846, 153.6272566616697191 ) ) ;
#11501=DIRECTION ( 'NONE',  ( 1.000000000000000000, 0.000000000000000000, 0.000000000000000000 ) ) ;
#11507=ORIENTED_EDGE ( 'NONE', *, *, #9208, .F. ) ;
#11510=AXIS2_PLACEMENT_3D ( 'NONE', #1542, #36429, #33231 ) ;
#11547=EDGE_CURVE ( 'NONE', #24301, #3405, #990, .T. ) ;
#11557=CARTESIAN_POINT ( 'NONE',  ( 1.261328688602779469, 4.650731711012212166, 153.0204462508474990 ) ) ;
#11563=ORIENTED_EDGE ( 'NONE', *, *, #13440, .T. ) ;
#11600=AXIS2_PLACEMENT_3D ( 'NONE', #3112, #39037, #13506 ) ;
#11629=ADVANCED_FACE ( 'NONE', ( #6937 ), #26937, .F. ) ;
#11636=DIRECTION ( 'NONE',  ( 0.8825449026266889430, 0.4702281306426152052, -0.000000000000000000 ) ) ;
#11650=VERTEX_POINT ( 'NONE', #20547 ) ;
#11664=DIRECTION ( 'NONE',  ( 0.000000000000000000, 0.000000000000000000, -1.000000000000000000 ) ) ;
#11667=ORIENTED_EDGE ( 'NONE', *, *, #17404, .F. ) ;
#11668=FACE_OUTER_BOUND ( 'NONE', #19603, .T. ) ;
#11670=CIRCLE ( 'NONE', #25966, 7.579174044925158782 ) ;
#11677=ORIENTED_EDGE ( 'NONE', *, *, #35088, .T. ) ;
#11688=CARTESIAN_POINT ( 'NONE',  ( 8.698099397114690490, 8.075154377652495441, 152.9676766984442793 ) ) ;
#11703=DIRECTION ( 'NONE',  ( -0.000000000000000000, -0.000000000000000000, -1.000000000000000000 ) ) ;
#11716=ORIENTED_EDGE ( 'NONE', *, *, #20756, .T. ) ;
#11755=LINE ( 'NONE', #38131, #39422 ) ;
#11762=CARTESIAN_POINT ( 'NONE',  ( 3.216997096249633703, 3.872784298312517137, 153.6940457802679703 ) ) ;
#11769=CARTESIAN_POINT ( 'NONE',  ( 0.5127800862017841688, 4.761333394820713494, 152.9200730884599579 ) ) ;
#11772=ORIENTED_EDGE ( 'NONE', *, *, #10261, .T. ) ;
#11787=AXIS2_PLACEMENT_3D ( 'NONE', #4182, #24964, #40120 ) ;
#11801=CARTESIAN_POINT ( 'NONE',  ( 3.742640687119171083, 20.81551514656773705, 159.5815388724490163 ) ) ;
#11811=ORIENTED_EDGE ( 'NONE', *, *, #11348, .T. ) ;
#11847=CARTESIAN_POINT ( 'NONE',  ( 9.718734271691502613, 23.11111384794381252, 159.5815388724490163 ) ) ;
#11854=DIRECTION ( 'NONE',  ( -1.000000000000000000, 0.000000000000000000, 0.000000000000000000 ) ) ;
#11859=CARTESIAN_POINT ( 'NONE',  ( 8.654913651897858884, 27.20455347664128354, 153.0774312600619567 ) ) ;
#11877=CARTESIAN_POINT ( 'NONE',  ( 0.6348918613210261519, 6.257764873244187065, 151.9983627981024767 ) ) ;
#11887=CARTESIAN_POINT ( 'NONE',  ( -2.604869650104253420, 31.41246745148119857, 159.5815388724490163 ) ) ;
#11901=CARTESIAN_POINT ( 'NONE',  ( 6.689291174884115954, 5.289692763229563610, 153.6451024763360635 ) ) ;
#11904=CARTESIAN_POINT ( 'NONE',  ( 4.330127018922107496, 20.00000000000014211, 155.5815388724490163 ) ) ;
#11909=EDGE_CURVE ( 'NONE', #21748, #27996, #30748, .T. ) ;
#11926=ORIENTED_EDGE ( 'NONE', *, *, #14525, .F. ) ;
#11940=EDGE_LOOP ( 'NONE', ( #30562, #9468, #32845, #34022 ) ) ;
#11948=SHAPE_REPRESENTATION_RELATIONSHIP ( 'NONE' , 'NONE' ,  #19321, #10203 ) ;
#11960=DIRECTION ( 'NONE',  ( 0.000000000000000000, -1.000000000000000000, 0.000000000000000000 ) ) ;
#12031=ORIENTED_EDGE ( 'NONE', *, *, #18806, .F. ) ;
#12058=DIRECTION ( 'NONE',  ( 1.000000000000000000, 0.000000000000000000, 0.000000000000000000 ) ) ;
#12062=DIRECTION ( 'NONE',  ( 0.000000000000000000, 0.000000000000000000, 1.000000000000000000 ) ) ;
#12068=ORIENTED_EDGE ( 'NONE', *, *, #10953, .F. ) ;
#12079=DIRECTION ( 'NONE',  ( -0.000000000000000000, -0.000000000000000000, -1.000000000000000000 ) ) ;
#12081=ORIENTED_EDGE ( 'NONE', *, *, #10319, .T. ) ;
#12087=CARTESIAN_POINT ( 'NONE',  ( 10.53587323178443569, 12.57181129186098723, 154.5815388724490163 ) ) ;
#12143=B_SPLINE_CURVE_WITH_KNOTS ( 'NONE', 3,
 ( #36410, #4507, #23663, #17897, #30871, #17488, #1733, #7488, #10679, #20248, #33852, #36625, #27057, #4713, #30660, #30450 ),
 .UNSPECIFIED., .F., .F.,
 ( 4, 2, 2, 2, 2, 2, 2, 4 ),
 ( 2.540748634419633256E-07, 0.001910996430635734629, 0.002866367608521882930, 0.003821738786408031014, 0.004777109964294178231, 0.005732481142180326748, 0.006687852320066474399, 0.007643223497952622916 ),
 .UNSPECIFIED. ) ;
#12151=EDGE_LOOP ( 'NONE', ( #1237, #36311 ) ) ;
#12170=ORIENTED_EDGE ( 'NONE', *, *, #20269, .T. ) ;
#12172=CARTESIAN_POINT ( 'NONE',  ( 1.000000000000119460, 6.211512421032414188, 154.5815388724490163 ) ) ;
#12192=EDGE_LOOP ( 'NONE', ( #40085, #10360, #10794, #30471 ) ) ;
#12193=ADVANCED_FACE ( 'NONE', ( #22424 ), #36232, .F. ) ;
#12199=CARTESIAN_POINT ( 'NONE',  ( 12.27165144158600185, 20.46975685308311554, 152.8454421597756436 ) ) ;
#12228=AXIS2_PLACEMENT_3D ( 'NONE', #29857, #33254, #4336 ) ;
#12237=CARTESIAN_POINT ( 'NONE',  ( 10.03587323178420476, 23.29421411192385349, 159.5815388724490163 ) ) ;
#12251=DIRECTION ( 'NONE',  ( 0.03404294460294553931, -0.9994203709764779564, 0.000000000000000000 ) ) ;
#12255=EDGE_CURVE ( 'NONE', #18108, #10736, #35429, .T. ) ;
#12271=DIRECTION ( 'NONE',  ( -0.000000000000000000, 0.000000000000000000, -1.000000000000000000 ) ) ;
#12280=ORIENTED_EDGE ( 'NONE', *, *, #22299, .T. ) ;
#12295=CARTESIAN_POINT ( 'NONE',  ( -3.563940842959833599, 29.61244032134267101, 152.8454421597756152 ) ) ;
#12303=AXIS2_PLACEMENT_3D ( 'NONE', #16724, #23317, #23097 ) ;
#12325=VECTOR ( 'NONE', #20861, 1000.000000000000000 ) ;
#12381=CARTESIAN_POINT ( 'NONE',  ( -16.28249153430137852, 26.90070087040669478, 159.5815388724490163 ) ) ;
#12400=CARTESIAN_POINT ( 'NONE',  ( 6.303637636350541307, 3.592856506039595832, 154.4788437011423810 ) ) ;
#12406=VECTOR ( 'NONE', #39283, 1000.000000000000000 ) ;
#12414=CARTESIAN_POINT ( 'NONE',  ( 12.51091437391554173, 20.32053375938133399, 152.9675281823368209 ) ) ;
#12420=B_SPLINE_CURVE_WITH_KNOTS ( 'NONE', 3,
 ( #10886, #23871, #20244, #13860, #20669, #40436, #30017, #23214, #20876, #30444, #10675, #33424, #33648, #17270, #3864, #30233, #36181, #11098, #40228, #33847, #39586, #10461, #4502, #33205, #29805, #23657 ),
 .UNSPECIFIED., .F., .F.,
 ( 4, 2, 2, 2, 2, 2, 2, 2, 2, 2, 2, 2, 4 ),
 ( 2.125331784252702803E-07, 0.001294100106468041699, 0.001941043893112849236, 0.002587987679757657207, 0.003234931466402464744, 0.003881875253047271847, 0.005175762826336885621, 0.006469650399626499827, 0.007116594186271311268, 0.007763537972916120973, 0.008410481759560930679, 0.009057425546205741251, 0.01035131311949533985 ),
 .UNSPECIFIED. ) ;
#12450=ORIENTED_EDGE ( 'NONE', *, *, #11377, .T. ) ;
#12461=EDGE_LOOP ( 'NONE', ( #8071, #25749, #32342, #16278 ) ) ;
#12470=DIRECTION ( 'NONE',  ( -1.000000000000000000, 0.000000000000000000, 0.000000000000000000 ) ) ;
#12472=DIRECTION ( 'NONE',  ( -0.000000000000000000, -0.000000000000000000, -1.000000000000000000 ) ) ;
#12486=DIRECTION ( 'NONE',  ( -0.000000000000000000, -0.000000000000000000, -1.000000000000000000 ) ) ;
#12487=CARTESIAN_POINT ( 'NONE',  ( -9.414900485372523775, 23.67904455026975441, 151.9992203709526848 ) ) ;
#12512=CARTESIAN_POINT ( 'NONE',  ( -16.28249153430137852, 26.90070087040669478, 154.5815388724490163 ) ) ;
#12517=CARTESIAN_POINT ( 'NONE',  ( -5.079011605969801835, 30.02419470480434782, 153.3946900320997031 ) ) ;
#12525=AXIS2_PLACEMENT_3D ( 'NONE', #11031, #10814, #36765 ) ;
#12535=LINE ( 'NONE', #28903, #21391 ) ;
#12545=CARTESIAN_POINT ( 'NONE',  ( -12.27165144158654719, 14.53024314691597141, 159.5815388724490163 ) ) ;
#12565=CIRCLE ( 'NONE', #18677, 11.07917404492516233 ) ;
#12594=ADVANCED_FACE ( 'NONE', ( #31434 ), #37004, .F. ) ;
#12613=CARTESIAN_POINT ( 'NONE',  ( 9.626159306789590531, 6.122734998444764543, 154.2527048017825848 ) ) ;
#12627=DIRECTION ( 'NONE',  ( 0.000000000000000000, 0.000000000000000000, -1.000000000000000000 ) ) ;
#12648=ADVANCED_FACE ( 'NONE', ( #9531 ), #41870, .T. ) ;
#12665=MECHANICAL_DESIGN_GEOMETRIC_PRESENTATION_REPRESENTATION('',(#35757),#4522);
#12673=ORIENTED_EDGE ( 'NONE', *, *, #3676, .T. ) ;
#12674=PRODUCT_CONTEXT ( 'NONE', #23372, 'mechanical' ) ;
#12676=ORIENTED_EDGE ( 'NONE', *, *, #16344, .F. ) ;
#12727=CARTESIAN_POINT ( 'NONE',  ( -3.302902078253353135, 29.47335644018510692, 152.7173827288297048 ) ) ;
#12731=ORIENTED_EDGE ( 'NONE', *, *, #841, .T. ) ;
#12735=CARTESIAN_POINT ( 'NONE',  ( -16.28249153430137497, 8.099299129593275026, 150.5815388724490163 ) ) ;
#12743=CARTESIAN_POINT ( 'NONE',  ( 8.892120608938066439, 29.91268222665748411, 154.4788437280928122 ) ) ;
#12772=VERTEX_POINT ( 'NONE', #6120 ) ;
#12788=CIRCLE ( 'NONE', #27732, 5.000000000000004441 ) ;
#12802=CARTESIAN_POINT ( 'NONE',  ( 10.41947860041720908, 17.49999999999956302, 159.5815388724490163 ) ) ;
#12819=CARTESIAN_POINT ( 'NONE',  ( 10.20684115509134315, 8.306252114835304567, 153.5324451153152836 ) ) ;
#12868=ORIENTED_EDGE ( 'NONE', *, *, #24044, .T. ) ;
#12933=CARTESIAN_POINT ( 'NONE',  ( -6.926659451089422603, 31.23917086733601423, 154.5487360771605836 ) ) ;
#12936=CARTESIAN_POINT ( 'NONE',  ( -5.381645978142303832, 4.977543395646510049, 153.4658060357146496 ) ) ;
#12941=ADVANCED_FACE ( 'NONE', ( #28350 ), #5385, .T. ) ;
#12948=CARTESIAN_POINT ( 'NONE',  ( 13.38682700280543436, 15.63811396994896974, 153.3951907928777700 ) ) ;
#12992=VECTOR ( 'NONE', #33262, 1000.000000000000000 ) ;
#13006=EDGE_CURVE ( 'NONE', #32814, #29598, #22771, .T. ) ;
#13025=FACE_OUTER_BOUND ( 'NONE', #59, .T. ) ;
#13033=EDGE_CURVE ( 'NONE', #9177, #2489, #11670, .T. ) ;
#13036=CARTESIAN_POINT ( 'NONE',  ( 10.58060021645987092, 24.77746367793933402, 152.9774433574588386 ) ) ;
#13037=AXIS2_PLACEMENT_3D ( 'NONE', #28019, #12271, #34195 ) ;
#13068=CARTESIAN_POINT ( 'NONE',  ( -9.718734271691911175, 23.11111384794358514, 154.5815388724490163 ) ) ;
#13103=CIRCLE ( 'NONE', #7005, 5.000000000000004441 ) ;
#13115=CARTESIAN_POINT ( 'NONE',  ( -10.27611701369020381, 22.27821838569869684, 159.5815388724490163 ) ) ;
#13125=CYLINDRICAL_SURFACE ( 'NONE', #16665, 5.000000000000000888 ) ;
#13138=CARTESIAN_POINT ( 'NONE',  ( -10.12905004066251280, 27.50877633989744808, 153.8406025264450250 ) ) ;
#13151=AXIS2_PLACEMENT_3D ( 'NONE', #1592, #13934, #17128 ) ;
#13182=CARTESIAN_POINT ( 'NONE',  ( -0.5127800862019271655, 30.23866660517787963, 152.9200730884596453 ) ) ;
#13189=ORIENTED_EDGE ( 'NONE', *, *, #13201, .T. ) ;
#13191=AXIS2_PLACEMENT_3D ( 'NONE', #28434, #41423, #18869 ) ;
#13196=DIRECTION ( 'NONE',  ( -1.000000000000000000, 0.000000000000000000, -0.000000000000000000 ) ) ;
#13201=EDGE_CURVE ( 'NONE', #29296, #12772, #21802, .T. ) ;
#13202=VERTEX_POINT ( 'NONE', #41374 ) ;
#13214=SPHERICAL_SURFACE ( 'NONE', #31305, 5.000000000000000000 ) ;
#13217=LINE ( 'NONE', #25780, #9689 ) ;
#13258=CARTESIAN_POINT ( 'NONE',  ( 8.707710598625942211, 26.64268346825921085, 159.5815388724490163 ) ) ;
#13268=FACE_OUTER_BOUND ( 'NONE', #30944, .T. ) ;
#13294=ORIENTED_EDGE ( 'NONE', *, *, #23105, .T. ) ;
#13295=AXIS2_PLACEMENT_3D ( 'NONE', #18227, #34596, #37583 ) ;
#13297=ORIENTED_EDGE ( 'NONE', *, *, #2308, .F. ) ;
#13300=VERTEX_POINT ( 'NONE', #18822 ) ;
#13302=CARTESIAN_POINT ( 'NONE',  ( -9.718734271691911175, 23.11111384794358514, 159.5815388724490163 ) ) ;
#13308=EDGE_LOOP ( 'NONE', ( #32684, #7128, #7916, #9757 ) ) ;
#13338=CARTESIAN_POINT ( 'NONE',  ( 2.302507646137074410E-15, -1.301401740813418195, 159.5815388724490163 ) ) ;
#13348=CARTESIAN_POINT ( 'NONE',  ( -4.822789029776409997, 31.51296647551156482, 154.2011256547282585 ) ) ;
#13358=VERTEX_POINT ( 'NONE', #15433 ) ;
#13359=( LENGTH_UNIT ( ) NAMED_UNIT ( * ) SI_UNIT ( .MILLI., .METRE. ) );
#13368=LINE ( 'NONE', #19964, #9440 ) ;
#13379=DIRECTION ( 'NONE',  ( -0.000000000000000000, -0.000000000000000000, -1.000000000000000000 ) ) ;
#13391=B_SPLINE_CURVE_WITH_KNOTS ( 'NONE', 3,
 ( #577, #25702, #38666, #42077, #22494, #13348, #16143, #35476, #19938, #39495, #38876, #12933, #6336, #26330, #25911, #19310, #36093, #32286, #6962, #9751, #22712, #32903, #29285, #13138, #29715, #13549 ),
 .UNSPECIFIED., .F., .F.,
 ( 4, 2, 2, 2, 2, 2, 2, 2, 2, 2, 2, 2, 4 ),
 ( 2.406822060242567640E-07, 0.001294128252029388970, 0.001941072036941073747, 0.002588015821852758091, 0.003234959606764442868, 0.003881903391676128079, 0.005175790961499497633, 0.006469678531322861983, 0.007116622316234537220, 0.007763566101146212456, 0.008410509886057888559, 0.009057453670969562928, 0.01035134124079288044 ),
 .UNSPECIFIED. ) ;
#13422=DIRECTION ( 'NONE',  ( 0.000000000000000000, 0.000000000000000000, 1.000000000000000000 ) ) ;
#13440=EDGE_CURVE ( 'NONE', #9160, #5451, #27970, .T. ) ;
#13485=EDGE_CURVE ( 'NONE', #8278, #1899, #5515, .T. ) ;
#13501=CIRCLE ( 'NONE', #25058, 7.579174044924941178 ) ;
#13506=DIRECTION ( 'NONE',  ( -0.5291922403339061054, 0.8485019580238937209, 0.000000000000000000 ) ) ;
#13532=CARTESIAN_POINT ( 'NONE',  ( 4.742640687119343390, 15.91653566100140615, 155.5815388724490163 ) ) ;
#13535=CIRCLE ( 'NONE', #8109, 7.579174044926197062 ) ;
#13544=PLANE ( 'NONE',  #27894 ) ;
#13549=CARTESIAN_POINT ( 'NONE',  ( -10.20684115509089906, 26.69374788516367403, 153.5324451153149994 ) ) ;
#13562=VERTEX_POINT ( 'NONE', #13068 ) ;
#13603=ORIENTED_EDGE ( 'NONE', *, *, #3993, .T. ) ;
#13619=ORIENTED_EDGE ( 'NONE', *, *, #9232, .F. ) ;
#13648=EDGE_LOOP ( 'NONE', ( #9195, #32972, #11366, #33151 ) ) ;
#13651=CARTESIAN_POINT ( 'NONE',  ( 4.643803883590850390, 29.98060070181117709, 153.2720928744884361 ) ) ;
#13670=DIRECTION ( 'NONE',  ( -1.000000000000000000, 0.000000000000000000, 0.000000000000000000 ) ) ;
#13711=CARTESIAN_POINT ( 'NONE',  ( -13.38787894130420497, 15.63974124508996866, 153.3956926483660368 ) ) ;
#13719=VERTEX_POINT ( 'NONE', #17399 ) ;
#13755=CARTESIAN_POINT ( 'NONE',  ( -13.03350328710566153, 19.83188372073434991, 153.2251063045277704 ) ) ;
#13762=ORIENTED_EDGE ( 'NONE', *, *, #39884, .F. ) ;
#13766=CARTESIAN_POINT ( 'NONE',  ( -10.27611701369020381, 22.27821838569869684, 154.5815388724490163 ) ) ;
#13777=CARTESIAN_POINT ( 'NONE',  ( -8.698099397114209097, 26.92484562234621848, 152.9676766984439666 ) ) ;
#13805=CARTESIAN_POINT ( 'NONE',  ( 0.000000000000000000, 36.30140174081339666, 159.5815388724490163 ) ) ;
#13820=CARTESIAN_POINT ( 'NONE',  ( 1.008723249705561598, 30.30116904610835604, 152.9768715499299390 ) ) ;
#13821=ORIENTED_EDGE ( 'NONE', *, *, #5964, .T. ) ;
#13822=CARTESIAN_POINT ( 'NONE',  ( 3.742640687119171083, 20.81551514656773705, 154.5815388724490163 ) ) ;
#13824=ORIENTED_EDGE ( 'NONE', *, *, #30262, .T. ) ;
#13860=CARTESIAN_POINT ( 'NONE',  ( -9.959961196147016693, 6.902270929826299195, 154.0304304313993384 ) ) ;
#13865=CARTESIAN_POINT ( 'NONE',  ( 5.209739300208924284, 8.476466837849169877, 164.5815388724490163 ) ) ;
#13880=EDGE_LOOP ( 'NONE', ( #17598, #30985, #40645, #38712 ) ) ;
#13890=AXIS2_PLACEMENT_3D ( 'NONE', #15479, #38223, #12058 ) ;
#13922=CARTESIAN_POINT ( 'NONE',  ( -13.76250257119345122, 16.45250485984112743, 153.5723417271109099 ) ) ;
#13934=DIRECTION ( 'NONE',  ( 0.000000000000000000, 0.000000000000000000, -1.000000000000000000 ) ) ;
#13995=EDGE_LOOP ( 'NONE', ( #39594, #21308, #4183, #36513 ) ) ;
#14001=EDGE_CURVE ( 'NONE', #29125, #29981, #170, .T. ) ;
#14002=ORIENTED_EDGE ( 'NONE', *, *, #26765, .F. ) ;
#14011=B_SPLINE_CURVE_WITH_KNOTS ( 'NONE', 3,
 ( #28667, #16556, #19316, #32291, #29508, #41659, #12517, #29086, #378, #25500, #6128, #9328, #35268, #19109, #32074, #2943, #28881, #41878, #23353, #585, #17393, #33555, #20366, #40138, #13777, #4416 ),
 .UNSPECIFIED., .F., .F.,
 ( 4, 2, 2, 2, 2, 2, 2, 2, 2, 2, 2, 2, 4 ),
 ( 2.437304301985370558E-07, 0.0009105819918572139165, 0.001365751122570733628, 0.001820920253284253340, 0.002276089383997773052, 0.002731258514711292981, 0.003641596776138325466, 0.004551935037565357084, 0.005007104168278871809, 0.005462273298992387401, 0.005917442429705902993, 0.006372611560419417717, 0.007282949821846422880 ),
 .UNSPECIFIED. ) ;
#14017=CARTESIAN_POINT ( 'NONE',  ( -10.20684115509165224, 8.306252114835197986, 159.5815388724490163 ) ) ;
#14021=DIRECTION ( 'NONE',  ( -0.000000000000000000, 0.000000000000000000, 1.000000000000000000 ) ) ;
#14023=CARTESIAN_POINT ( 'NONE',  ( -15.97057991159785217, 17.49999999999956657, 154.9135024962512546 ) ) ;
#14025=DIRECTION ( 'NONE',  ( -0.000000000000000000, -0.000000000000000000, -1.000000000000000000 ) ) ;
#14026=DIRECTION ( 'NONE',  ( 0.000000000000000000, 0.000000000000000000, -1.000000000000000000 ) ) ;
#14057=ORIENTED_EDGE ( 'NONE', *, *, #40727, .T. ) ;
#14076=CARTESIAN_POINT ( 'NONE',  ( 2.858598646995990755, 4.063742324715650334, 150.5815388724490163 ) ) ;
#14091=ORIENTED_EDGE ( 'NONE', *, *, #35265, .F. ) ;
#14096=ADVANCED_FACE ( 'NONE', ( #34386 ), #22245, .F. ) ;
#14121=CARTESIAN_POINT ( 'NONE',  ( -12.66641187784915701, 12.99212775466049230, 153.3506918906572594 ) ) ;
#14134=CARTESIAN_POINT ( 'NONE',  ( -13.59976475949396679, 16.03091716902233799, 153.4960580910870078 ) ) ;
#14137=EDGE_LOOP ( 'NONE', ( #37172, #22563, #7290, #12068, #33591, #856, #2742, #41065 ) ) ;
#14140=ORIENTED_EDGE ( 'NONE', *, *, #11909, .F. ) ;
#14149=DIRECTION ( 'NONE',  ( -0.000000000000000000, -0.000000000000000000, 1.000000000000000000 ) ) ;
#14171=ADVANCED_FACE ( 'NONE', ( #29237 ), #23292, .F. ) ;
#14205=VERTEX_POINT ( 'NONE', #39445 ) ;
#14241=EDGE_CURVE ( 'NONE', #13562, #38421, #9918, .T. ) ;
#14245=DIRECTION ( 'NONE',  ( -0.000000000000000000, -0.000000000000000000, 1.000000000000000000 ) ) ;
#14283=EDGE_CURVE ( 'NONE', #21985, #19992, #16706, .T. ) ;
#14292=DIRECTION ( 'NONE',  ( 0.8660254037844397068, -0.4999999999999979461, 0.000000000000000000 ) ) ;
#14311=CARTESIAN_POINT ( 'NONE',  ( 16.28249153430138207, 8.099299129593287461, 164.5815388724490163 ) ) ;
#14347=CARTESIAN_POINT ( 'NONE',  ( -2.429273991871403915, 4.276629443760617377, 153.3506918668365699 ) ) ;
#14356=DIRECTION ( 'NONE',  ( 0.000000000000000000, -0.000000000000000000, -1.000000000000000000 ) ) ;
#14368=DIRECTION ( 'NONE',  ( 1.000000000000000000, 0.000000000000000000, 0.000000000000000000 ) ) ;
#14372=B_SPLINE_CURVE_WITH_KNOTS ( 'NONE', 3,
 ( #3603, #39764, #22756, #35931, #6795, #13182, #6381, #22538, #23172, #13820, #7011, #39540, #6593, #39323, #10204, #19988 ),
 .UNSPECIFIED., .F., .F.,
 ( 4, 2, 2, 2, 2, 2, 2, 4 ),
 ( 2.411650883979177127E-07, 0.001523416315041781601, 0.002285003890018463737, 0.003046591464995146090, 0.003808179039971828876, 0.004569766614948511663, 0.005331354189925195317, 0.006092941764901877236 ),
 .UNSPECIFIED. ) ;
#14406=DIRECTION ( 'NONE',  ( -1.000000000000000000, 0.000000000000000000, 0.000000000000000000 ) ) ;
#14425=AXIS2_PLACEMENT_3D ( 'NONE', #2302, #18256, #15290 ) ;
#14462=VERTEX_POINT ( 'NONE', #36907 ) ;
#14471=EDGE_CURVE ( 'NONE', #9150, #20191, #854, .T. ) ;
#14486=DIRECTION ( 'NONE',  ( -1.000000000000000000, 0.000000000000000000, 0.000000000000000000 ) ) ;
#14509=CARTESIAN_POINT ( 'NONE',  ( 7.229790860939806940, 29.39824960736702764, 153.6451024802794620 ) ) ;
#14522=DIRECTION ( 'NONE',  ( -0.000000000000000000, -0.000000000000000000, -1.000000000000000000 ) ) ;
#14525=EDGE_CURVE ( 'NONE', #10845, #14205, #29769, .T. ) ;
#14542=CARTESIAN_POINT ( 'NONE',  ( 16.28249153430137852, 26.90070087040669122, 159.5815388724490163 ) ) ;
#14543=AXIS2_PLACEMENT_3D ( 'NONE', #13338, #6952, #36296 ) ;
#14555=CIRCLE ( 'NONE', #19315, 3.500000000000003997 ) ;
#14575=ORIENTED_EDGE ( 'NONE', *, *, #9324, .F. ) ;
#14579=CARTESIAN_POINT ( 'NONE',  ( 5.209739300208926061, 8.476466837849169877, 159.5815388724490163 ) ) ;
#14606=DIRECTION ( 'NONE',  ( 0.5000000000000038858, -0.8660254037844363761, 0.000000000000000000 ) ) ;
#14618=ORIENTED_EDGE ( 'NONE', *, *, #24128, .F. ) ;
#14621=ORIENTED_EDGE ( 'NONE', *, *, #32656, .T. ) ;
#14629=B_SPLINE_CURVE_WITH_KNOTS ( 'NONE', 3,
 ( #21558, #5391, #10944, #11557, #23928, #11769, #17954, #7760, #36898, #14770, #24549, #17746, #1788, #14347, #8166, #1372 ),
 .UNSPECIFIED., .F., .F.,
 ( 4, 2, 2, 2, 2, 2, 2, 4 ),
 ( 2.411650883963629837E-07, 0.001523416315041857712, 0.002285003890018588637, 0.003046591464995319128, 0.003808179039972049620, 0.004569766614948781412, 0.005331354189925511904, 0.006092941764902242395 ),
 .UNSPECIFIED. ) ;
#14630=LINE ( 'NONE', #11421, #26904 ) ;
#14647=CARTESIAN_POINT ( 'NONE',  ( -16.28249153430137497, 8.099299129593275026, 159.5815388724490163 ) ) ;
#14660=DIRECTION ( 'NONE',  ( -0.000000000000000000, 0.000000000000000000, 1.000000000000000000 ) ) ;
#14666=FACE_OUTER_BOUND ( 'NONE', #37431, .T. ) ;
#14667=CARTESIAN_POINT ( 'NONE',  ( -1.196959198423996895E-13, 22.49999999999999289, 155.5815388724490163 ) ) ;
#14668=EDGE_LOOP ( 'NONE', ( #17323, #11563, #37166, #8803 ) ) ;
#14696=CARTESIAN_POINT ( 'NONE',  ( 8.153942370607722978, 6.578129285979470886, 153.4658061086812779 ) ) ;
#14704=DIRECTION ( 'NONE',  ( -0.8825449026267040420, 0.4702281306425870055, -0.000000000000000000 ) ) ;
#14726=DIRECTION ( 'NONE',  ( 1.000000000000000000, 0.000000000000000000, 0.000000000000000000 ) ) ;
#14737=ORIENTED_EDGE ( 'NONE', *, *, #33128, .F. ) ;
#14741=( NAMED_UNIT ( * ) SI_UNIT ( $, .STERADIAN. ) SOLID_ANGLE_UNIT ( ) );
#14770=CARTESIAN_POINT ( 'NONE',  ( -1.008723249705788527, 4.698830953890169582, 152.9768715499303937 ) ) ;
#14784=DIRECTION ( 'NONE',  ( -0.000000000000000000, 0.000000000000000000, 1.000000000000000000 ) ) ;
#14845=FACE_OUTER_BOUND ( 'NONE', #21774, .T. ) ;
#14905=DIRECTION ( 'NONE',  ( -0.4999999999999979461, -0.8660254037844397068, 0.000000000000000000 ) ) ;
#14909=LINE ( 'NONE', #21703, #21333 ) ;
#14951=EDGE_CURVE ( 'NONE', #6544, #8699, #10480, .T. ) ;
#14953=CARTESIAN_POINT ( 'NONE',  ( 1.000000000000119460, 5.911571776152701574, 159.5815388724490163 ) ) ;
#14966=CARTESIAN_POINT ( 'NONE',  ( 8.083882785676493654, 4.361833438080393144, 154.5729385747530671 ) ) ;
#14968=CARTESIAN_POINT ( 'NONE',  ( 0.000000000000000000, 17.49999999999998934, 141.5815388724490163 ) ) ;
#14993=CARTESIAN_POINT ( 'NONE',  ( -16.28249153430137852, 26.90070087040669478, 164.5815388724490163 ) ) ;
#15031=ORIENTED_EDGE ( 'NONE', *, *, #20722, .F. ) ;
#15033=CIRCLE ( 'NONE', #29287, 7.579174044926336506 ) ;
#15034=CARTESIAN_POINT ( 'NONE',  ( 5.209739300208269697, 26.52353316214887613, 159.5815388724490163 ) ) ;
#15040=ORIENTED_EDGE ( 'NONE', *, *, #14471, .T. ) ;
#15041=CARTESIAN_POINT ( 'NONE',  ( -14.54810494377379193, 14.67180503597531072, 154.2016150273003916 ) ) ;
#15044=AXIS2_PLACEMENT_3D ( 'NONE', #6258, #9449, #32816 ) ;
#15070=FACE_OUTER_BOUND ( 'NONE', #24135, .T. ) ;
#15080=CARTESIAN_POINT ( 'NONE',  ( -1.578877475748253989, 6.118048602964601734, 152.1415020100059792 ) ) ;
#15083=ORIENTED_EDGE ( 'NONE', *, *, #31934, .F. ) ;
#15106=CARTESIAN_POINT ( 'NONE',  ( 3.563940842959894884, 5.387559678655694739, 152.8454421597760700 ) ) ;
#15110=VECTOR ( 'NONE', #25155, 1000.000000000000000 ) ;
#15125=CARTESIAN_POINT ( 'NONE',  ( 5.000000000000004441, 17.49999999999998934, 155.5815388724490163 ) ) ;
#15135=LINE ( 'NONE', #24298, #35346 ) ;
#15143=ORIENTED_EDGE ( 'NONE', *, *, #14241, .T. ) ;
#15163=CARTESIAN_POINT ( 'NONE',  ( 13.06543980208709499, 13.25749020988031823, 153.5324451153150562 ) ) ;
#15170=DIRECTION ( 'NONE',  ( 1.000000000000000000, 0.000000000000000000, 0.000000000000000000 ) ) ;
#15172=VERTEX_POINT ( 'NONE', #37683 ) ;
#15176=DIRECTION ( 'NONE',  ( -0.000000000000000000, -0.000000000000000000, -1.000000000000000000 ) ) ;
#15211=EDGE_CURVE ( 'NONE', #6594, #9816, #8540, .T. ) ;
#15218=DIRECTION ( 'NONE',  ( 0.000000000000000000, 0.000000000000000000, 1.000000000000000000 ) ) ;
#15268=DIRECTION ( 'NONE',  ( 0.4702281306426152052, -0.8825449026266888319, 0.000000000000000000 ) ) ;
#15270=CARTESIAN_POINT ( 'NONE',  ( 0.000000000000000000, 36.30140174081339666, 150.5815388724490163 ) ) ;
#15279=FACE_OUTER_BOUND ( 'NONE', #37812, .T. ) ;
#15281=CIRCLE ( 'NONE', #3719, 5.000000000000004441 ) ;
#15290=DIRECTION ( 'NONE',  ( 0.8660254037844432595, -0.4999999999999918954, 0.000000000000000000 ) ) ;
#15294=CARTESIAN_POINT ( 'NONE',  ( 1.268010732602645518, 28.82242955212867486, 152.0807008677961960 ) ) ;
#15301=ORIENTED_EDGE ( 'NONE', *, *, #16249, .T. ) ;
#15313=ORIENTED_EDGE ( 'NONE', *, *, #685, .F. ) ;
#15324=CARTESIAN_POINT ( 'NONE',  ( 5.521922812467409791, 4.987180720715727489, 153.4949357518737258 ) ) ;
#15339=FACE_OUTER_BOUND ( 'NONE', #25561, .T. ) ;
#15345=VECTOR ( 'NONE', #31217, 1000.000000000000000 ) ;
#15370=ORIENTED_EDGE ( 'NONE', *, *, #24044, .F. ) ;
#15373=CIRCLE ( 'NONE', #13295, 7.579174044925959919 ) ;
#15392=DIRECTION ( 'NONE',  ( -0.000000000000000000, 0.000000000000000000, 1.000000000000000000 ) ) ;
#15433=CARTESIAN_POINT ( 'NONE',  ( 5.000000000000004441, 17.49999999999998934, 141.5815388724490163 ) ) ;
#15458=ORIENTED_EDGE ( 'NONE', *, *, #33598, .F. ) ;
#15479=CARTESIAN_POINT ( 'NONE',  ( 16.28249153430137852, 26.90070087040669122, 164.5815388724490163 ) ) ;
#15490=PLANE ( 'NONE',  #23769 ) ;
#15554=DIRECTION ( 'NONE',  ( -0.000000000000000000, -0.000000000000000000, -1.000000000000000000 ) ) ;
#15562=EDGE_CURVE ( 'NONE', #6544, #40091, #859, .T. ) ;
#15565=ADVANCED_FACE ( 'NONE', ( #37018 ), #7665, .T. ) ;
#15580=CIRCLE ( 'NONE', #28467, 7.579174044926336506 ) ;
#15586=CARTESIAN_POINT ( 'NONE',  ( 14.66328716377125474, 14.84773288080794629, 154.2514967876345224 ) ) ;
#15589=B_SPLINE_CURVE_WITH_KNOTS ( 'NONE', 3,
 ( #35275, #19532, #31868, #22726, #6138, #9973, #12948, #38678, #35703, #29302, #15941, #6567, #32503, #6352 ),
 .UNSPECIFIED., .F., .F.,
 ( 4, 2, 2, 2, 2, 2, 4 ),
 ( 2.534995935963242109E-07, 0.0009116973918458201641, 0.001367419337971934002, 0.001823141284098047732, 0.002278863230224153005, 0.002734585176350258062, 0.003646029068602458199 ),
 .UNSPECIFIED. ) ;
#15594=PLANE ( 'NONE',  #25386 ) ;
#15601=CARTESIAN_POINT ( 'NONE',  ( 3.596493781833070891, 3.725862423057630934, 153.8381731320200743 ) ) ;
#15636=LINE ( 'NONE', #39204, #24820 ) ;
#15661=VERTEX_POINT ( 'NONE', #17240 ) ;
#15674=CARTESIAN_POINT ( 'NONE',  ( 10.03587323178444279, 11.70578588807654441, 159.5815388724490163 ) ) ;
#15687=DIRECTION ( 'NONE',  ( -0.000000000000000000, -0.000000000000000000, -1.000000000000000000 ) ) ;
#15712=CARTESIAN_POINT ( 'NONE',  ( -8.698105546967914492, 8.075334922794642267, 152.9675984850773602 ) ) ;
#15715=CARTESIAN_POINT ( 'NONE',  ( 0.3107243566307155702, 6.278133426388396110, 151.9771749059764829 ) ) ;
#15717=ORIENTED_EDGE ( 'NONE', *, *, #28217, .F. ) ;
#15722=CYLINDRICAL_SURFACE ( 'NONE', #31941, 6.079174044925164111 ) ;
#15741=EDGE_CURVE ( 'NONE', #37916, #30300, #200, .T. ) ;
#15746=CYLINDRICAL_SURFACE ( 'NONE', #28072, 7.579174044926197062 ) ;
#15788=AXIS2_PLACEMENT_3D ( 'NONE', #22586, #34929, #15799 ) ;
#15794=DIRECTION ( 'NONE',  ( -1.000000000000000000, 0.000000000000000000, 0.000000000000000000 ) ) ;
#15799=DIRECTION ( 'NONE',  ( -1.000000000000000000, 0.000000000000000000, 0.000000000000000000 ) ) ;
#15808=DIRECTION ( 'NONE',  ( -0.5000000000000101030, 0.8660254037844328234, 0.000000000000000000 ) ) ;
#15810=ORIENTED_EDGE ( 'NONE', *, *, #1751, .F. ) ;
#15832=EDGE_CURVE ( 'NONE', #5194, #1623, #25354, .T. ) ;
#15866=EDGE_LOOP ( 'NONE', ( #18589, #25036, #10007, #27798, #41726, #25537, #15040, #28835, #10021, #27978, #32032, #19260, #3257, #38469, #12170, #33962 ) ) ;
#15904=CARTESIAN_POINT ( 'NONE',  ( -8.707710598626182019, 26.64268346825927836, 152.8454421597756436 ) ) ;
#15930=CARTESIAN_POINT ( 'NONE',  ( -7.791185372434255463, 6.108136644985679098, 153.5717503904285479 ) ) ;
#15931=ORIENTED_EDGE ( 'NONE', *, *, #4675, .F. ) ;
#15934=CARTESIAN_POINT ( 'NONE',  ( -0.6437596841452616347, 6.256934695609817965, 151.9992204069324657 ) ) ;
#15937=ORIENTED_EDGE ( 'NONE', *, *, #8177, .F. ) ;
#15941=CARTESIAN_POINT ( 'NONE',  ( 13.76218140321552674, 16.45155205783633789, 153.5721917427163419 ) ) ;
#15949=CARTESIAN_POINT ( 'NONE',  ( 8.435140907414792721, 30.36824880957956196, 154.5487361196971108 ) ) ;
#15986=CIRCLE ( 'NONE', #20746, 7.579174044924941178 ) ;
#15991=EDGE_CURVE ( 'NONE', #11650, #10845, #15589, .T. ) ;
#16007=DIRECTION ( 'NONE',  ( 0.000000000000000000, 1.000000000000000000, 0.000000000000000000 ) ) ;
#16032=CARTESIAN_POINT ( 'NONE',  ( 10.12905004066307413, 7.491223660101412385, 153.8406025264453660 ) ) ;
#16055=APPLICATION_CONTEXT ( 'automotive_design' ) ;
#16076=ADVANCED_FACE ( 'NONE', ( #41886 ), #15722, .F. ) ;
#16114=LINE ( 'NONE', #9723, #9118 ) ;
#16119=CARTESIAN_POINT ( 'NONE',  ( -12.02068193548590713, 20.62628108255945136, 152.7173827546451719 ) ) ;
#16143=CARTESIAN_POINT ( 'NONE',  ( -5.032437754690646692, 31.52482352993746773, 154.2509714831750216 ) ) ;
#16146=CARTESIAN_POINT ( 'NONE',  ( -6.417378831302253062, 5.177370420822439812, 153.6272566164931277 ) ) ;
#16166=EDGE_CURVE ( 'NONE', #13358, #19992, #17020, .T. ) ;
#16217=CARTESIAN_POINT ( 'NONE',  ( -9.535873231784242066, 10.83976048429175520, 159.5815388724490163 ) ) ;
#16243=CARTESIAN_POINT ( 'NONE',  ( -13.06543980208727262, 21.74250979011898721, 153.5324451153151983 ) ) ;
#16249=EDGE_CURVE ( 'NONE', #15661, #27377, #15135, .T. ) ;
#16278=ORIENTED_EDGE ( 'NONE', *, *, #35986, .T. ) ;
#16280=ADVANCED_FACE ( 'NONE', ( #17907 ), #18316, .F. ) ;
#16291=ORIENTED_EDGE ( 'NONE', *, *, #39731, .F. ) ;
#16325=CARTESIAN_POINT ( 'NONE',  ( 10.20684115509134315, 8.306252114835304567, 153.5324451153152836 ) ) ;
#16344=EDGE_CURVE ( 'NONE', #35681, #5552, #30884, .T. ) ;
#16345=CARTESIAN_POINT ( 'NONE',  ( -7.470466625469991406, 5.787504423504878481, 153.6264001176294869 ) ) ;
#16354=FACE_OUTER_BOUND ( 'NONE', #21714, .T. ) ;
#16364=CARTESIAN_POINT ( 'NONE',  ( 9.959961196145831863, 28.09772907017222821, 154.0304304313984858 ) ) ;
#16412=VECTOR ( 'NONE', #24265, 1000.000000000000000 ) ;
#16433=ORIENTED_EDGE ( 'NONE', *, *, #12255, .T. ) ;
#16435=DIRECTION ( 'NONE',  ( -1.000000000000000000, 0.000000000000000000, 0.000000000000000000 ) ) ;
#16437=CARTESIAN_POINT ( 'NONE',  ( 9.411389837927153224, 5.757836299279407655, 154.3424624685366666 ) ) ;
#16456=VECTOR ( 'NONE', #34988, 999.9999999999998863 ) ;
#16490=VECTOR ( 'NONE', #19267, 1000.000000000000000 ) ;
#16493=LINE ( 'NONE', #29442, #29809 ) ;
#16512=EDGE_CURVE ( 'NONE', #20517, #3564, #19369, .T. ) ;
#16515=DIRECTION ( 'NONE',  ( -0.8660254037844397068, 0.4999999999999979461, 0.000000000000000000 ) ) ;
#16522=PLANE ( 'NONE',  #12303 ) ;
#16523=PRODUCT_DEFINITION_CONTEXT ( 'detailed design', #16055, 'design' ) ;
#16532=CARTESIAN_POINT ( 'NONE',  ( 10.89329215898968783, 10.92378321506238059, 152.9047840745571136 ) ) ;
#16556=CARTESIAN_POINT ( 'NONE',  ( -3.812946306956360942, 29.74511274798788207, 152.9675983386008511 ) ) ;
#16559=CIRCLE ( 'NONE', #7716, 7.579174044925959919 ) ;
#16571=CIRCLE ( 'NONE', #24050, 6.079174044925482967 ) ;
#16572=CARTESIAN_POINT ( 'NONE',  ( 6.098656404397392095, 31.44852239414950290, 154.4507088739389360 ) ) ;
#16609=ORIENTED_EDGE ( 'NONE', *, *, #11296, .T. ) ;
#16665=AXIS2_PLACEMENT_3D ( 'NONE', #355, #32271, #22480 ) ;
#16687=CARTESIAN_POINT ( 'NONE',  ( -5.209739300209236035, 8.476466837849001124, 159.5815388724490163 ) ) ;
#16698=CARTESIAN_POINT ( 'NONE',  ( -12.73537588372967555, 14.86005412084119470, 153.0791759260053766 ) ) ;
#16706=LINE ( 'NONE', #19674, #18516 ) ;
#16710=EDGE_LOOP ( 'NONE', ( #39506, #4683, #22672, #20304, #8903, #29398, #3241, #25218, #36376, #13297, #33604, #36778, #26753, #23989, #29340, #12450 ) ) ;
#16724=CARTESIAN_POINT ( 'NONE',  ( -1.000000000000119460, 29.08842822384727356, 154.5815388724490163 ) ) ;
#16753=ADVANCED_FACE ( 'NONE', ( #3049 ), #9865, .T. ) ;
#16759=VERTEX_POINT ( 'NONE', #25811 ) ;
#16784=CARTESIAN_POINT ( 'NONE',  ( 9.276117013689805901, 24.01026919326780629, 154.5815388724490163 ) ) ;
#16788=DIRECTION ( 'NONE',  ( -1.000000000000000000, 0.000000000000000000, -0.000000000000000000 ) ) ;
#16857=ORIENTED_EDGE ( 'NONE', *, *, #31923, .T. ) ;
#16911=ORIENTED_EDGE ( 'NONE', *, *, #33968, .F. ) ;
#16932=UNCERTAINTY_MEASURE_WITH_UNIT (LENGTH_MEASURE( 1.000000000000000082E-05 ), #11327, 'distance_accuracy_value', 'NONE');
#16959=CARTESIAN_POINT ( 'NONE',  ( 5.209739300208926949, 8.476466837849169877, 159.5815388724490163 ) ) ;
#16970=VERTEX_POINT ( 'NONE', #34594 ) ;
#16971=EDGE_LOOP ( 'NONE', ( #35841, #5080, #11716, #20689 ) ) ;
#17009=CARTESIAN_POINT ( 'NONE',  ( -5.209739300209232482, 8.476466837849001124, 159.5815388724490163 ) ) ;
#17020=CIRCLE ( 'NONE', #18345, 5.000000000000004441 ) ;
#17068=CARTESIAN_POINT ( 'NONE',  ( 12.66641187784861522, 22.00787224533859643, 153.3506918906570036 ) ) ;
#17128=DIRECTION ( 'NONE',  ( -1.000000000000000000, 0.000000000000000000, 0.000000000000000000 ) ) ;
#17139=DIRECTION ( 'NONE',  ( 0.000000000000000000, -0.000000000000000000, -1.000000000000000000 ) ) ;
#17153=AXIS2_PLACEMENT_3D ( 'NONE', #18692, #34636, #35062 ) ;
#17172=ADVANCED_FACE ( 'NONE', ( #18225 ), #25456, .T. ) ;
#17176=DIRECTION ( 'NONE',  ( 0.000000000000000000, 1.000000000000000000, 0.000000000000000000 ) ) ;
#17188=CYLINDRICAL_SURFACE ( 'NONE', #9261, 6.079174044925482967 ) ;
#17240=CARTESIAN_POINT ( 'NONE',  ( 9.718734271692364146, 11.88888615205621946, 154.5815388724490163 ) ) ;
#17270=CARTESIAN_POINT ( 'NONE',  ( -7.336044244482998522, 3.930068663829043185, 154.5729385715628155 ) ) ;
#17276=CARTESIAN_POINT ( 'NONE',  ( 5.209739300208926061, 8.476466837849169877, 159.5815388724490163 ) ) ;
#17306=EDGE_CURVE ( 'NONE', #5451, #13300, #6828, .T. ) ;
#17315=CIRCLE ( 'NONE', #41081, 3.500000000000001332 ) ;
#17319=CARTESIAN_POINT ( 'NONE',  ( -11.14181700333092273, 11.35424083990906929, 152.9047840894036199 ) ) ;
#17323=ORIENTED_EDGE ( 'NONE', *, *, #35286, .F. ) ;
#17331=CARTESIAN_POINT ( 'NONE',  ( -13.91947860041774909, 17.19286710119477846, 153.6452861111158654 ) ) ;
#17339=VERTEX_POINT ( 'NONE', #35846 ) ;
#17353=DIRECTION ( 'NONE',  ( 0.4999999999999980016, 0.8660254037844398178, 0.000000000000000000 ) ) ;
#17393=CARTESIAN_POINT ( 'NONE',  ( -8.371260436319985843, 28.03230184839122785, 153.3570253316110552 ) ) ;
#17399=CARTESIAN_POINT ( 'NONE',  ( -1.000000000000119460, 22.39897948556632201, 154.5815388724490163 ) ) ;
#17404=EDGE_CURVE ( 'NONE', #13202, #11324, #36262, .T. ) ;
#17406=CARTESIAN_POINT ( 'NONE',  ( -15.36256818513920130, 18.36675792270974128, 154.5490570889041635 ) ) ;
#17433=ORIENTED_EDGE ( 'NONE', *, *, #18048, .F. ) ;
#17485=CARTESIAN_POINT ( 'NONE',  ( 15.15544456622768621, 8.750000000000028422, 154.5815388724490163 ) ) ;
#17487=ORIENTED_EDGE ( 'NONE', *, *, #31923, .F. ) ;
#17488=CARTESIAN_POINT ( 'NONE',  ( 10.05866016940721863, 22.56402018877686544, 151.9992204325093894 ) ) ;
#17489=CARTESIAN_POINT ( 'NONE',  ( 5.530144355237426979, 30.01206074506895405, 153.4965619403743915 ) ) ;
#17502=CARTESIAN_POINT ( 'NONE',  ( -11.75845712892207118, 22.83229142561944158, 153.0204462570418968 ) ) ;
#17525=CARTESIAN_POINT ( 'NONE',  ( -10.20684115509165224, 8.306252114835194433, 153.5324451153154826 ) ) ;
#17555=ORIENTED_EDGE ( 'NONE', *, *, #8691, .T. ) ;
#17565=EDGE_CURVE ( 'NONE', #27996, #28419, #10915, .T. ) ;
#17572=DIRECTION ( 'NONE',  ( -0.000000000000000000, -0.000000000000000000, -1.000000000000000000 ) ) ;
#17596=EDGE_LOOP ( 'NONE', ( #6013, #2106, #28969, #11772 ) ) ;
#17598=ORIENTED_EDGE ( 'NONE', *, *, #7793, .F. ) ;
#17600=VERTEX_POINT ( 'NONE', #1178 ) ;
#17607=DIRECTION ( 'NONE',  ( 1.000000000000000000, 0.000000000000000000, 0.000000000000000000 ) ) ;
#17612=CARTESIAN_POINT ( 'NONE',  ( -15.12727392775299684, 19.19785311792891491, 154.4499356296062729 ) ) ;
#17616=CARTESIAN_POINT ( 'NONE',  ( -1.000000000000119460, 29.08842822384727356, 154.5815388724490163 ) ) ;
#17647=EDGE_LOOP ( 'NONE', ( #33559, #12031, #34417, #2146 ) ) ;
#17704=EDGE_LOOP ( 'NONE', ( #2564, #13821, #19198, #37735 ) ) ;
#17707=CARTESIAN_POINT ( 'NONE',  ( 12.27165144158615107, 14.53024314691610819, 159.5815388724490163 ) ) ;
#17733=CARTESIAN_POINT ( 'NONE',  ( 9.535873231784194104, 24.16023951570828032, 154.5815388724490163 ) ) ;
#17746=CARTESIAN_POINT ( 'NONE',  ( -1.737309318840124961, 4.529558681323030633, 153.1288291135480506 ) ) ;
#17770=B_SPLINE_CURVE_WITH_KNOTS ( 'NONE', 3,
 ( #28029, #41008, #11859, #37814, #20886, #7918, #33857, #27276, #4718, #30666, #11109, #1531, #14509, #4508, #10466, #7278, #3871, #17489, #27476, #26631, #23877, #13651, #27272, #36626, #39817, #37059 ),
 .UNSPECIFIED., .F., .F.,
 ( 4, 2, 2, 2, 2, 2, 2, 2, 2, 2, 2, 2, 4 ),
 ( 2.152236452720500467E-07, 0.0009105534912595450144, 0.001365722625066699558, 0.001820891758873854427, 0.002276060892681009296, 0.002731230026488163515, 0.003641568294102481926, 0.004551906561716800338, 0.005007075695523955858, 0.005462244829331110510, 0.005917413963138265162, 0.006372583096945420682, 0.007282921364559755140 ),
 .UNSPECIFIED. ) ;
#17805=ORIENTED_EDGE ( 'NONE', *, *, #35547, .T. ) ;
#17806=ADVANCED_FACE ( 'NONE', ( #9013 ), #38154, .T. ) ;
#17814=CARTESIAN_POINT ( 'NONE',  ( -15.41947860041774376, 17.49999999999956657, 154.5727510624246293 ) ) ;
#17874=DIRECTION ( 'NONE',  ( 0.03404294460277332984, 0.9994203709764838406, -0.000000000000000000 ) ) ;
#17897=CARTESIAN_POINT ( 'NONE',  ( 10.64649782989203075, 21.82362765082753953, 152.1415020206850954 ) ) ;
#17899=ORIENTED_EDGE ( 'NONE', *, *, #11296, .F. ) ;
#17901=FACE_OUTER_BOUND ( 'NONE', #35375, .T. ) ;
#17905=CARTESIAN_POINT ( 'NONE',  ( 13.06543980208691913, 21.74250979011892326, 159.5815388724490163 ) ) ;
#17907=FACE_OUTER_BOUND ( 'NONE', #30179, .T. ) ;
#17912=DIRECTION ( 'NONE',  ( -0.000000000000000000, -0.000000000000000000, -1.000000000000000000 ) ) ;
#17923=( NAMED_UNIT ( * ) PLANE_ANGLE_UNIT ( ) SI_UNIT ( $, .RADIAN. ) );
#17948=DIRECTION ( 'NONE',  ( 0.8660254037844328234, 0.5000000000000101030, 0.000000000000000000 ) ) ;
#17951=DIRECTION ( 'NONE',  ( 1.000000000000000000, 0.000000000000000000, 0.000000000000000000 ) ) ;
#17954=CARTESIAN_POINT ( 'NONE',  ( 0.2606827522252246898, 4.777514670994612800, 152.9052493585882075 ) ) ;
#17956=ORIENTED_EDGE ( 'NONE', *, *, #39719, .F. ) ;
#17970=FACE_OUTER_BOUND ( 'NONE', #29874, .T. ) ;
#17971=VECTOR ( 'NONE', #32370, 999.9999999999998863 ) ;
#18005=EDGE_LOOP ( 'NONE', ( #14091, #19053, #21527 ) ) ;
#18034=CYLINDRICAL_SURFACE ( 'NONE', #36792, 7.579174044925158782 ) ;
#18048=EDGE_CURVE ( 'NONE', #9150, #28722, #9870, .T. ) ;
#18086=CARTESIAN_POINT ( 'NONE',  ( 8.653841190006842155, 7.790126473778983929, 153.0794454334391901 ) ) ;
#18092=VECTOR ( 'NONE', #41667, 1000.000000000000000 ) ;
#18096=CARTESIAN_POINT ( 'NONE',  ( -1.196959198423996895E-13, 22.49999999999999289, 154.5815388724490163 ) ) ;
#18108=VERTEX_POINT ( 'NONE', #33448 ) ;
#18121=ORIENTED_EDGE ( 'NONE', *, *, #21747, .T. ) ;
#18143=DIRECTION ( 'NONE',  ( 1.000000000000000000, 0.000000000000000000, 0.000000000000000000 ) ) ;
#18154=EDGE_CURVE ( 'NONE', #29981, #4657, #10235, .T. ) ;
#18178=DIRECTION ( 'NONE',  ( -0.000000000000000000, -0.000000000000000000, -1.000000000000000000 ) ) ;
#18225=FACE_OUTER_BOUND ( 'NONE', #12192, .T. ) ;
#18227=CARTESIAN_POINT ( 'NONE',  ( -16.28249153430137852, 26.90070087040669478, 159.5815388724490163 ) ) ;
#18245=CARTESIAN_POINT ( 'NONE',  ( 4.330127018922280691, 15.00000000000012967, 155.5815388724490163 ) ) ;
#18256=DIRECTION ( 'NONE',  ( -0.4999999999999919509, -0.8660254037844433705, 0.000000000000000000 ) ) ;
#18272=EDGE_LOOP ( 'NONE', ( #12673, #2377, #751, #1992 ) ) ;
#18287=CARTESIAN_POINT ( 'NONE',  ( 4.496074243414229343, 5.046971837806230710, 153.2247034038996674 ) ) ;
#18290=LINE ( 'NONE', #11904, #19213 ) ;
#18299=ADVANCED_FACE ( 'NONE', ( #23735 ), #7563, .F. ) ;
#18312=CARTESIAN_POINT ( 'NONE',  ( 1.000000000000119460, 6.211512421032414188, 159.5815388724490163 ) ) ;
#18316=PLANE ( 'NONE',  #22443 ) ;
#18343=CARTESIAN_POINT ( 'NONE',  ( 10.20684115509066103, 26.69374788516360297, 150.5815388724490163 ) ) ;
#18345=AXIS2_PLACEMENT_3D ( 'NONE', #40655, #27890, #14726 ) ;
#18377=CARTESIAN_POINT ( 'NONE',  ( 13.53450912783508464, 19.10266903390744275, 153.4652957816659580 ) ) ;
#18385=DIRECTION ( 'NONE',  ( -1.000000000000000000, 0.000000000000000000, 0.000000000000000000 ) ) ;
#18402=EDGE_CURVE ( 'NONE', #4657, #13300, #21812, .T. ) ;
#18414=EDGE_CURVE ( 'NONE', #3157, #645, #20958, .T. ) ;
#18420=DIRECTION ( 'NONE',  ( -1.000000000000000000, 0.000000000000000000, 0.000000000000000000 ) ) ;
#18422=VERTEX_POINT ( 'NONE', #21578 ) ;
#18459=VERTEX_POINT ( 'NONE', #18605 ) ;
#18474=ORIENTED_EDGE ( 'NONE', *, *, #30025, .F. ) ;
#18476=CARTESIAN_POINT ( 'NONE',  ( 2.468635207678250953, 5.870845545476611527, 152.3877646471614753 ) ) ;
#18478=EDGE_LOOP ( 'NONE', ( #32915, #8421, #33058, #13603 ) ) ;
#18480=LINE ( 'NONE', #12087, #18092 ) ;
#18516=VECTOR ( 'NONE', #32646, 1000.000000000000000 ) ;
#18559=FACE_OUTER_BOUND ( 'NONE', #18005, .T. ) ;
#18589=ORIENTED_EDGE ( 'NONE', *, *, #21514, .T. ) ;
#18605=CARTESIAN_POINT ( 'NONE',  ( 4.742640687119343390, 15.91653566100140615, 159.5815388724490163 ) ) ;
#18650=VERTEX_POINT ( 'NONE', #24992 ) ;
#18652=CARTESIAN_POINT ( 'NONE',  ( -13.06543980208746092, 13.25749020988016547, 153.5324451153153120 ) ) ;
#18662=AXIS2_PLACEMENT_3D ( 'NONE', #7891, #33833, #4691 ) ;
#18677=AXIS2_PLACEMENT_3D ( 'NONE', #9441, #6250, #22409 ) ;
#18692=CARTESIAN_POINT ( 'NONE',  ( -10.41947860041774199, 17.49999999999951683, 159.5815388724490163 ) ) ;
#18731=ORIENTED_EDGE ( 'NONE', *, *, #6102, .T. ) ;
#18747=ADVANCED_FACE ( 'NONE', ( #38847 ), #16522, .F. ) ;
#18754=ORIENTED_EDGE ( 'NONE', *, *, #18154, .T. ) ;
#18755=DIRECTION ( 'NONE',  ( -0.000000000000000000, -0.000000000000000000, 1.000000000000000000 ) ) ;
#18787=CARTESIAN_POINT ( 'NONE',  ( 6.089894672131651809, 3.549879163702124085, 154.4494414891316865 ) ) ;
#18798=CARTESIAN_POINT ( 'NONE',  ( 13.30584406242254225, 19.48505323181119664, 153.3565333127145607 ) ) ;
#18806=EDGE_CURVE ( 'NONE', #21263, #10573, #36494, .T. ) ;
#18822=CARTESIAN_POINT ( 'NONE',  ( -10.41947860041774199, 17.49999999999951683, 164.5815388724490163 ) ) ;
#18837=EDGE_CURVE ( 'NONE', #19636, #20517, #7990, .T. ) ;
#18841=ORIENTED_EDGE ( 'NONE', *, *, #24857, .F. ) ;
#18842=VERTEX_POINT ( 'NONE', #39894 ) ;
#18854=CARTESIAN_POINT ( 'NONE',  ( -15.12794563354735189, 15.80414247959125262, 154.4502191185283380 ) ) ;
#18866=CARTESIAN_POINT ( 'NONE',  ( 2.858598646995994308, 4.063742324715648557, 153.5324451153153973 ) ) ;
#18869=DIRECTION ( 'NONE',  ( -1.000000000000000000, 0.000000000000000000, 0.000000000000000000 ) ) ;
#18893=CARTESIAN_POINT ( 'NONE',  ( -8.075457743341729611, 6.461464625110996174, 153.4949358233103851 ) ) ;
#18896=DIRECTION ( 'NONE',  ( -0.000000000000000000, 0.000000000000000000, 1.000000000000000000 ) ) ;
#18945=CIRCLE ( 'NONE', #39297, 5.000000000000000000 ) ;
#19000=ORIENTED_EDGE ( 'NONE', *, *, #24877, .F. ) ;
#19004=AXIS2_PLACEMENT_3D ( 'NONE', #2076, #41004, #11854 ) ;
#19027=DIRECTION ( 'NONE',  ( -1.000000000000000000, 0.000000000000000000, 0.000000000000000000 ) ) ;
#19053=ORIENTED_EDGE ( 'NONE', *, *, #29231, .T. ) ;
#19062=ORIENTED_EDGE ( 'NONE', *, *, #32452, .F. ) ;
#19076=VECTOR ( 'NONE', #25663, 1000.000000000000114 ) ;
#19106=CARTESIAN_POINT ( 'NONE',  ( -2.468635207678232746, 29.12915445452188479, 152.3877646471609921 ) ) ;
#19107=EDGE_CURVE ( 'NONE', #2489, #12772, #28791, .T. ) ;
#19109=CARTESIAN_POINT ( 'NONE',  ( -7.222421200248130724, 29.40341411833024310, 153.6454670892161403 ) ) ;
#19123=B_SPLINE_CURVE_WITH_KNOTS ( 'NONE', 3,
 ( #15904, #35666, #32466, #6313, #32262, #12487, #2915, #32669, #22470, #25472, #28851, #3129, #133, #9729, #16119, #29060 ),
 .UNSPECIFIED., .F., .F.,
 ( 4, 2, 2, 2, 2, 2, 2, 4 ),
 ( 2.157098444381531571E-07, 0.001910958079630901843, 0.002866329264524129089, 0.003821700449417356985, 0.004777071634310584881, 0.005732442819203811477, 0.006687814004097039806, 0.007643185188990267269 ),
 .UNSPECIFIED. ) ;
#19124=ADVANCED_FACE ( 'NONE', ( #13268 ), #32664, .T. ) ;
#19188=CARTESIAN_POINT ( 'NONE',  ( 14.15884394889443421, 14.17435182453268716, 154.0308563845580920 ) ) ;
#19198=ORIENTED_EDGE ( 'NONE', *, *, #27690, .F. ) ;
#19203=CARTESIAN_POINT ( 'NONE',  ( -16.28249153430137497, 8.099299129593275026, 159.5815388724490163 ) ) ;
#19213=VECTOR ( 'NONE', #6161, 1000.000000000000000 ) ;
#19222=DIRECTION ( 'NONE',  ( -0.000000000000000000, -0.000000000000000000, -1.000000000000000000 ) ) ;
#19225=CARTESIAN_POINT ( 'NONE',  ( -13.91947860041774376, 17.49999999999951683, 159.5815388724490163 ) ) ;
#19260=ORIENTED_EDGE ( 'NONE', *, *, #24650, .F. ) ;
#19267=DIRECTION ( 'NONE',  ( 0.000000000000000000, 0.000000000000000000, 1.000000000000000000 ) ) ;
#19268=CARTESIAN_POINT ( 'NONE',  ( -10.41947860041774199, 17.49999999999951683, 159.5815388724490163 ) ) ;
#19277=CIRCLE ( 'NONE', #41688, 5.000000000000004441 ) ;
#19294=CARTESIAN_POINT ( 'NONE',  ( 14.16111231062217612, 20.82305157546459995, 154.0318591658866012 ) ) ;
#19301=ORIENTED_EDGE ( 'NONE', *, *, #25136, .F. ) ;
#19310=CARTESIAN_POINT ( 'NONE',  ( -8.886277873992222354, 29.91908985729988402, 154.4799523825321046 ) ) ;
#19315=AXIS2_PLACEMENT_3D ( 'NONE', #37773, #8628, #5863 ) ;
#19316=CARTESIAN_POINT ( 'NONE',  ( -4.076932598375554662, 29.84765169955398889, 153.0774311017628690 ) ) ;
#19321=SHAPE_REPRESENTATION ( 'Long Screw Plastic Knob - Handle', ( #40442 ), #38405 ) ;
#19324=CIRCLE ( 'NONE', #13191, 7.579174044926197062 ) ;
#19331=AXIS2_PLACEMENT_3D ( 'NONE', #14311, #27290, #39836 ) ;
#19332=CARTESIAN_POINT ( 'NONE',  ( 10.19301642060052160, 27.09960940607311386, 153.6940459180243010 ) ) ;
#19354=ORIENTED_EDGE ( 'NONE', *, *, #375, .F. ) ;
#19369=LINE ( 'NONE', #36534, #33316 ) ;
#19398=CARTESIAN_POINT ( 'NONE',  ( 4.330127018922280691, 15.00000000000012967, 154.5815388724490163 ) ) ;
#19422=ORIENTED_EDGE ( 'NONE', *, *, #2956, .T. ) ;
#19439=CARTESIAN_POINT ( 'NONE',  ( -9.276117013690740265, 10.98973080673171765, 159.5815388724490163 ) ) ;
#19463=ADVANCED_FACE ( 'NONE', ( #32152 ), #13214, .T. ) ;
#19502=CARTESIAN_POINT ( 'NONE',  ( 10.58177606127877191, 10.22583576541548744, 152.9768715113189899 ) ) ;
#19523=CARTESIAN_POINT ( 'NONE',  ( -4.643803883591428594, 5.019399298186760561, 153.2720928744893740 ) ) ;
#19532=CARTESIAN_POINT ( 'NONE',  ( 12.51134252589913132, 14.67973326970979109, 152.9677466506646510 ) ) ;
#19537=CARTESIAN_POINT ( 'NONE',  ( 7.336044244482061494, 31.06993133616881053, 154.5729385715619060 ) ) ;
#19578=EDGE_LOOP ( 'NONE', ( #11222, #24921, #26218, #41977 ) ) ;
#19594=LINE ( 'NONE', #16217, #17971 ) ;
#19603=EDGE_LOOP ( 'NONE', ( #13619, #9374, #10113, #22449 ) ) ;
#19608=CARTESIAN_POINT ( 'NONE',  ( 9.722444945200486188, 6.313176583623129723, 154.2021328665920521 ) ) ;
#19612=ORIENTED_EDGE ( 'NONE', *, *, #27179, .T. ) ;
#19636=VERTEX_POINT ( 'NONE', #10230 ) ;
#19652=CARTESIAN_POINT ( 'NONE',  ( -8.707710598626928089, 8.357316531739312992, 152.8454421597761836 ) ) ;
#19653=DIRECTION ( 'NONE',  ( 0.000000000000000000, 0.000000000000000000, -1.000000000000000000 ) ) ;
#19665=CARTESIAN_POINT ( 'NONE',  ( -13.87973638471602023, 16.89268013571968297, 153.6269493541827558 ) ) ;
#19674=CARTESIAN_POINT ( 'NONE',  ( -5.000000000000004441, 17.49999999999998934, 155.5815388724490163 ) ) ;
#19675=ADVANCED_FACE ( 'NONE', ( #7038 ), #26826, .F. ) ;
#19696=AXIS2_PLACEMENT_3D ( 'NONE', #17733, #7532, #24332 ) ;
#19738=EDGE_CURVE ( 'NONE', #18650, #6293, #39571, .T. ) ;
#19747=CARTESIAN_POINT ( 'NONE',  ( 9.036211638866731732, 29.74906396683514842, 154.4494414979802457 ) ) ;
#19769=CYLINDRICAL_SURFACE ( 'NONE', #2170, 3.500000000000003997 ) ;
#19779=ORIENTED_EDGE ( 'NONE', *, *, #33688, .F. ) ;
#19785=ORIENTED_EDGE ( 'NONE', *, *, #160, .T. ) ;
#19819=ORIENTED_EDGE ( 'NONE', *, *, #32993, .F. ) ;
#19825=CARTESIAN_POINT ( 'NONE',  ( 11.14181700333034541, 23.64575916008989509, 152.9047840894032504 ) ) ;
#19861=CARTESIAN_POINT ( 'NONE',  ( -8.717779811042197124, 8.652924803142948207, 152.7173826728528070 ) ) ;
#19862=CARTESIAN_POINT ( 'NONE',  ( -8.707710598626180243, 26.64268346825927836, 159.5815388724490163 ) ) ;
#19866=VERTEX_POINT ( 'NONE', #31055 ) ;
#19920=CARTESIAN_POINT ( 'NONE',  ( 12.27165144158615107, 14.53024314691610819, 159.5815388724490163 ) ) ;
#19938=CARTESIAN_POINT ( 'NONE',  ( -5.665064099548538401, 31.50736892558343882, 154.3802602213496300 ) ) ;
#19964=CARTESIAN_POINT ( 'NONE',  ( 10.20684115509134315, 8.306252114835304567, 150.5815388724490163 ) ) ;
#19973=CARTESIAN_POINT ( 'NONE',  ( -2.604869650104253420, 31.41246745148119857, 159.5815388724490163 ) ) ;
#19977=CARTESIAN_POINT ( 'NONE',  ( -13.06543980208746092, 13.25749020988016547, 153.5324451153153120 ) ) ;
#19988=CARTESIAN_POINT ( 'NONE',  ( 2.858598646995926362, 30.93625767528271098, 153.5324451153149141 ) ) ;
#19992=VERTEX_POINT ( 'NONE', #28065 ) ;
#19993=EDGE_CURVE ( 'NONE', #26392, #10736, #41046, .T. ) ;
#19996=VERTEX_POINT ( 'NONE', #37235 ) ;
#20041=ORIENTED_EDGE ( 'NONE', *, *, #34418, .T. ) ;
#20048=CARTESIAN_POINT ( 'NONE',  ( 11.28496987124398743, 23.43009685274535059, 152.9195735306842607 ) ) ;
#20052=ORIENTED_EDGE ( 'NONE', *, *, #15562, .T. ) ;
#20064=CIRCLE ( 'NONE', #32299, 5.000000000000001776 ) ;
#20093=CARTESIAN_POINT ( 'NONE',  ( -12.51091437391608352, 14.67946624061774230, 152.9675281823371904 ) ) ;
#20100=ORIENTED_EDGE ( 'NONE', *, *, #32455, .F. ) ;
#20191=VERTEX_POINT ( 'NONE', #20816 ) ;
#20209=ORIENTED_EDGE ( 'NONE', *, *, #9018, .T. ) ;
#20227=DIRECTION ( 'NONE',  ( -1.000000000000000000, 0.000000000000000000, 0.000000000000000000 ) ) ;
#20236=CARTESIAN_POINT ( 'NONE',  ( 8.727825599366525466, 8.947845398623483604, 152.5896210917541111 ) ) ;
#20244=CARTESIAN_POINT ( 'NONE',  ( -10.13050606591954050, 7.498275799549433351, 153.8381732780038931 ) ) ;
#20248=CARTESIAN_POINT ( 'NONE',  ( 9.173198941868744072, 24.25456285598690798, 152.0797565808655065 ) ) ;
#20256=CARTESIAN_POINT ( 'NONE',  ( 12.10138637141881901, 22.48066662991587705, 153.1288291267217971 ) ) ;
#20269=EDGE_CURVE ( 'NONE', #2094, #9007, #7609, .T. ) ;
#20292=ORIENTED_EDGE ( 'NONE', *, *, #37881, .F. ) ;
#20295=CARTESIAN_POINT ( 'NONE',  ( 3.742640687119171528, 20.81551514656774415, 155.5815388724490163 ) ) ;
#20304=ORIENTED_EDGE ( 'NONE', *, *, #35286, .T. ) ;
#20334=DIRECTION ( 'NONE',  ( 0.000000000000000000, 0.000000000000000000, 1.000000000000000000 ) ) ;
#20361=AXIS2_PLACEMENT_3D ( 'NONE', #31020, #14026, #4232 ) ;
#20366=CARTESIAN_POINT ( 'NONE',  ( -8.534991945851048811, 27.62508664397032732, 153.2263581680551852 ) ) ;
#20370=ORIENTED_EDGE ( 'NONE', *, *, #10854, .T. ) ;
#20375=VERTEX_POINT ( 'NONE', #1864 ) ;
#20414=VERTEX_POINT ( 'NONE', #22063 ) ;
#20417=ORIENTED_EDGE ( 'NONE', *, *, #6193, .F. ) ;
#20432=ORIENTED_EDGE ( 'NONE', *, *, #14241, .F. ) ;
#20443=DIRECTION ( 'NONE',  ( -0.000000000000000000, 0.000000000000000000, -1.000000000000000000 ) ) ;
#20449=CARTESIAN_POINT ( 'NONE',  ( 9.414900485372513117, 11.32095544972909629, 151.9992203709527985 ) ) ;
#20453=CARTESIAN_POINT ( 'NONE',  ( -12.27165144158644239, 20.46975685308312620, 152.8454421597758994 ) ) ;
#20471=ORIENTED_EDGE ( 'NONE', *, *, #3835, .T. ) ;
#20477=ADVANCED_FACE ( 'NONE', ( #37391 ), #18034, .T. ) ;
#20478=ORIENTED_EDGE ( 'NONE', *, *, #34230, .F. ) ;
#20517=VERTEX_POINT ( 'NONE', #32263 ) ;
#20542=DIRECTION ( 'NONE',  ( -0.000000000000000000, 1.000000000000000000, -0.000000000000000000 ) ) ;
#20547=CARTESIAN_POINT ( 'NONE',  ( 12.27165144158615284, 14.53024314691610641, 152.8454421597757289 ) ) ;
#20591=CARTESIAN_POINT ( 'NONE',  ( -13.06543980208727262, 21.74250979011898721, 153.5324451153151983 ) ) ;
#20615=CLOSED_SHELL ( 'NONE', ( #4630, #38351, #2311, #32955, #12648, #6714, #16753, #20477, #12941, #26239, #37899, #9626, #34969, #37362, #37637, #22745, #12193, #14096, #32840, #15565, #10875, #35739, #6764, #41362, #2604, #34019, #7923, #29453, #7940, #18747, #6236, #14171, #27751, #242, #23843, #12594, #31367, #23793, #16280, #36805, #28816, #11434, #23526, #19675, #18299, #719, #4434, #17806, #5779, #29534, #9229, #1782, #19124, #2653, #29513, #36609, #8562, #7742, #10059, #19463, #34961, #17172, #16076, #4257, #3071, #24059, #36932, #782, #38185, #23460, #3010, #11629 ) ) ;
#20644=ORIENTED_EDGE ( 'NONE', *, *, #18402, .T. ) ;
#20669=CARTESIAN_POINT ( 'NONE',  ( -9.889506012871194685, 6.703345612976963075, 154.0908813678220497 ) ) ;
#20689=ORIENTED_EDGE ( 'NONE', *, *, #31813, .F. ) ;
#20722=EDGE_CURVE ( 'NONE', #2257, #17339, #22526, .T. ) ;
#20733=LINE ( 'NONE', #24344, #31843 ) ;
#20746=AXIS2_PLACEMENT_3D ( 'NONE', #5846, #1609, #19027 ) ;
#20748=ORIENTED_EDGE ( 'NONE', *, *, #36015, .T. ) ;
#20756=EDGE_CURVE ( 'NONE', #37916, #8278, #40327, .T. ) ;
#20757=DIRECTION ( 'NONE',  ( 0.000000000000000000, -0.000000000000000000, -1.000000000000000000 ) ) ;
#20816=CARTESIAN_POINT ( 'NONE',  ( -4.330127018922262927, 19.99999999999987566, 154.5815388724490163 ) ) ;
#20833=DIRECTION ( 'NONE',  ( -1.000000000000000000, 0.000000000000000000, 0.000000000000000000 ) ) ;
#20846=DIRECTION ( 'NONE',  ( -1.000000000000000000, 0.000000000000000000, -0.000000000000000000 ) ) ;
#20861=DIRECTION ( 'NONE',  ( -0.000000000000000000, -0.000000000000000000, -1.000000000000000000 ) ) ;
#20876=CARTESIAN_POINT ( 'NONE',  ( -9.298205070446494247, 5.590225826412721588, 154.3802602823914754 ) ) ;
#20882=DIRECTION ( 'NONE',  ( -1.000000000000000000, 0.000000000000000000, 0.000000000000000000 ) ) ;
#20886=CARTESIAN_POINT ( 'NONE',  ( 8.487683822071625528, 27.75911101074991549, 153.2711608817832598 ) ) ;
#20925=B_SPLINE_CURVE_WITH_KNOTS ( 'NONE', 3,
 ( #15163, #23911, #7740, #19188, #8982, #6214, #15586, #31732, #35350, #2600, #22372, #32160, #2816, #3023 ),
 .UNSPECIFIED., .F., .F.,
 ( 4, 2, 2, 2, 2, 2, 4 ),
 ( 2.503320336978003087E-07, 0.001295412938146556225, 0.001942994241202997217, 0.002590575544259438208, 0.003238156847315879633, 0.003885738150372320624, 0.005180900756485223857 ),
 .UNSPECIFIED. ) ;
#20958=LINE ( 'NONE', #24787, #62 ) ;
#20962=CARTESIAN_POINT ( 'NONE',  ( -1.000000000000119460, 29.08842822384727356, 159.5815388724490163 ) ) ;
#20998=VERTEX_POINT ( 'NONE', #11801 ) ;
#21024=LINE ( 'NONE', #14023, #37060 ) ;
#21070=DIRECTION ( 'NONE',  ( -1.000000000000000000, 0.000000000000000000, 0.000000000000000000 ) ) ;
#21114=AXIS2_PLACEMENT_3D ( 'NONE', #29679, #17139, #32870 ) ;
#21136=CARTESIAN_POINT ( 'NONE',  ( 1.196959198423996895E-13, 5.911571776152701574, 159.5815388724490163 ) ) ;
#21139=CARTESIAN_POINT ( 'NONE',  ( -5.209739300208505952, 26.52353316214900047, 159.5815388724490163 ) ) ;
#21155=DIRECTION ( 'NONE',  ( 0.000000000000000000, 0.000000000000000000, -1.000000000000000000 ) ) ;
#21194=ORIENTED_EDGE ( 'NONE', *, *, #2308, .T. ) ;
#21202=ORIENTED_EDGE ( 'NONE', *, *, #31813, .T. ) ;
#21204=VECTOR ( 'NONE', #17572, 1000.000000000000000 ) ;
#21209=CARTESIAN_POINT ( 'NONE',  ( -13.91947860041774376, 17.49999999999951683, 153.6452861111158086 ) ) ;
#21215=AXIS2_PLACEMENT_3D ( 'NONE', #28044, #18896, #32075 ) ;
#21255=ORIENTED_EDGE ( 'NONE', *, *, #27567, .T. ) ;
#21263=VERTEX_POINT ( 'NONE', #40549 ) ;
#21296=VERTEX_POINT ( 'NONE', #1834 ) ;
#21299=ORIENTED_EDGE ( 'NONE', *, *, #2744, .T. ) ;
#21308=ORIENTED_EDGE ( 'NONE', *, *, #28041, .T. ) ;
#21333=VECTOR ( 'NONE', #2770, 1000.000000000000000 ) ;
#21391=VECTOR ( 'NONE', #5940, 1000.000000000000000 ) ;
#21409=DIRECTION ( 'NONE',  ( -1.000000000000000000, 0.000000000000000000, 0.000000000000000000 ) ) ;
#21417=CIRCLE ( 'NONE', #31591, 3.500000000000000444 ) ;
#21429=AXIS2_PLACEMENT_3D ( 'NONE', #6736, #32476, #10355 ) ;
#21430=CARTESIAN_POINT ( 'NONE',  ( -2.604869650104253420, 31.41246745148119857, 159.5815388724490163 ) ) ;
#21465=PLANE ( 'NONE',  #3061 ) ;
#21481=CARTESIAN_POINT ( 'NONE',  ( 4.932408324001740674, 4.984381444656370341, 153.3561522493817506 ) ) ;
#21484=CARTESIAN_POINT ( 'NONE',  ( 11.30546083962604520, 13.82332362234119749, 152.3877646696490444 ) ) ;
#21508=DIRECTION ( 'NONE',  ( -0.000000000000000000, -0.000000000000000000, -1.000000000000000000 ) ) ;
#21510=CARTESIAN_POINT ( 'NONE',  ( 10.20684115509134315, 8.306252114835304567, 153.5324451153152836 ) ) ;
#21514=EDGE_CURVE ( 'NONE', #37941, #32027, #2859, .T. ) ;
#21524=DIRECTION ( 'NONE',  ( 0.000000000000000000, 0.000000000000000000, 1.000000000000000000 ) ) ;
#21527=ORIENTED_EDGE ( 'NONE', *, *, #3854, .F. ) ;
#21542=DIRECTION ( 'NONE',  ( -0.000000000000000000, 0.000000000000000000, 1.000000000000000000 ) ) ;
#21558=CARTESIAN_POINT ( 'NONE',  ( 2.858598646995994308, 4.063742324715648557, 153.5324451153153973 ) ) ;
#21571=EDGE_CURVE ( 'NONE', #16759, #37941, #31595, .T. ) ;
#21578=CARTESIAN_POINT ( 'NONE',  ( 4.742640687119343390, 15.91653566100140615, 154.5815388724490163 ) ) ;
#21620=LINE ( 'NONE', #15674, #22826 ) ;
#21641=CIRCLE ( 'NONE', #6705, 3.500000000000001332 ) ;
#21643=DIRECTION ( 'NONE',  ( 0.4999999999999919509, 0.8660254037844433705, 0.000000000000000000 ) ) ;
#21655=LINE ( 'NONE', #14667, #32539 ) ;
#21658=CARTESIAN_POINT ( 'NONE',  ( 2.173728193257104646, 5.966035469847466466, 152.2937014792880177 ) ) ;
#21686=CARTESIAN_POINT ( 'NONE',  ( 4.076932598375653249, 5.152348300444276497, 153.0774311017634659 ) ) ;
#21698=CARTESIAN_POINT ( 'NONE',  ( 16.28249153430138207, 8.099299129593287461, 159.5815388724490163 ) ) ;
#21703=CARTESIAN_POINT ( 'NONE',  ( -12.27165144158644061, 20.46975685308312976, 159.5815388724490163 ) ) ;
#21714=EDGE_LOOP ( 'NONE', ( #26081, #20052, #19062, #12868 ) ) ;
#21715=VECTOR ( 'NONE', #11104, 1000.000000000000000 ) ;
#21747=EDGE_CURVE ( 'NONE', #15661, #8117, #29847, .T. ) ;
#21748=VERTEX_POINT ( 'NONE', #4094 ) ;
#21763=DIRECTION ( 'NONE',  ( 1.000000000000000000, 0.000000000000000000, -0.000000000000000000 ) ) ;
#21774=EDGE_LOOP ( 'NONE', ( #1954, #29937, #13762, #18731, #26469, #29551, #27737, #33127, #16291, #1780, #33329, #6288, #5758, #8642, #40867, #14057 ) ) ;
#21775=CARTESIAN_POINT ( 'NONE',  ( 13.76250257119291120, 18.54749514015794887, 153.5723417271105973 ) ) ;
#21802=LINE ( 'NONE', #5641, #16456 ) ;
#21812=CIRCLE ( 'NONE', #35413, 11.07917404492595814 ) ;
#21861=CARTESIAN_POINT ( 'NONE',  ( -9.718734271691911175, 23.11111384794358514, 159.5815388724490163 ) ) ;
#21907=AXIS2_PLACEMENT_3D ( 'NONE', #35432, #29880, #3510 ) ;
#21924=DIRECTION ( 'NONE',  ( 0.000000000000000000, -1.000000000000000000, 0.000000000000000000 ) ) ;
#21929=LINE ( 'NONE', #17707, #35031 ) ;
#21958=CARTESIAN_POINT ( 'NONE',  ( 10.53587323178443569, 12.57181129186098723, 159.5815388724490163 ) ) ;
#21968=VECTOR ( 'NONE', #6010, 999.9999999999998863 ) ;
#21972=FACE_BOUND ( 'NONE', #9096, .T. ) ;
#21985=VERTEX_POINT ( 'NONE', #594 ) ;
#21987=CARTESIAN_POINT ( 'NONE',  ( 13.03525533430953409, 19.82988963179798247, 153.2259575457066205 ) ) ;
#22031=CARTESIAN_POINT ( 'NONE',  ( -5.209739300208505064, 26.52353316214900047, 159.5815388724490163 ) ) ;
#22047=CARTESIAN_POINT ( 'NONE',  ( -15.36329688951122741, 16.63670233136802779, 154.5493626814887307 ) ) ;
#22063=CARTESIAN_POINT ( 'NONE',  ( 13.06543980208692091, 21.74250979011892326, 153.5324451153149710 ) ) ;
#22082=DIRECTION ( 'NONE',  ( -1.000000000000000000, 0.000000000000000000, 0.000000000000000000 ) ) ;
#22126=ORIENTED_EDGE ( 'NONE', *, *, #34009, .T. ) ;
#22228=EDGE_LOOP ( 'NONE', ( #18841, #35431, #1859, #25499, #35978, #24665, #31005, #30449 ) ) ;
#22235=CARTESIAN_POINT ( 'NONE',  ( 16.28249153430138207, 8.099299129593287461, 159.5815388724490163 ) ) ;
#22245=CYLINDRICAL_SURFACE ( 'NONE', #34817, 3.500000000000000444 ) ;
#22266=DIRECTION ( 'NONE',  ( 0.000000000000000000, 0.000000000000000000, 1.000000000000000000 ) ) ;
#22291=CARTESIAN_POINT ( 'NONE',  ( -1.570573766093413592, 28.88021343203565650, 152.1397377750288342 ) ) ;
#22299=EDGE_CURVE ( 'NONE', #9150, #13202, #33779, .T. ) ;
#22324=DIRECTION ( 'NONE',  ( -0.000000000000000000, -0.000000000000000000, -1.000000000000000000 ) ) ;
#22348=DIRECTION ( 'NONE',  ( 0.000000000000000000, 0.000000000000000000, -1.000000000000000000 ) ) ;
#22367=DIRECTION ( 'NONE',  ( 0.000000000000000000, 0.000000000000000000, -1.000000000000000000 ) ) ;
#22372=CARTESIAN_POINT ( 'NONE',  ( 15.19684507887511593, 16.00898674878502348, 154.4793021320810169 ) ) ;
#22380=CARTESIAN_POINT ( 'NONE',  ( -10.03587323178424562, 11.70578588807619091, 159.5815388724490163 ) ) ;
#22409=DIRECTION ( 'NONE',  ( 1.000000000000000000, -3.601228736517792616E-15, 0.000000000000000000 ) ) ;
#22424=FACE_OUTER_BOUND ( 'NONE', #29169, .T. ) ;
#22428=CARTESIAN_POINT ( 'NONE',  ( -11.77029632476451759, 14.21755885082801996, 152.5896212872840181 ) ) ;
#22443=AXIS2_PLACEMENT_3D ( 'NONE', #27488, #5557, #5139 ) ;
#22449=ORIENTED_EDGE ( 'NONE', *, *, #3676, .F. ) ;
#22470=CARTESIAN_POINT ( 'NONE',  ( -10.05350722043628764, 22.57128497180622873, 151.9983628076606976 ) ) ;
#22477=CARTESIAN_POINT ( 'NONE',  ( 14.96622041527852609, 19.59110817524664938, 154.3815176410579966 ) ) ;
#22480=DIRECTION ( 'NONE',  ( -1.000000000000000000, 0.000000000000000000, 0.000000000000000000 ) ) ;
#22494=CARTESIAN_POINT ( 'NONE',  ( -4.405423949752073298, 31.46289062211277709, 154.0908813598604183 ) ) ;
#22496=TOROIDAL_SURFACE ( 'NONE', #9598, 11.07917404492633828, 5.000000000000000000 ) ;
#22498=CARTESIAN_POINT ( 'NONE',  ( -8.707710598626928089, 8.357316531739312992, 152.8454421597761836 ) ) ;
#22514=CARTESIAN_POINT ( 'NONE',  ( 8.092379817708824419, 30.63221819749038133, 154.5725613230233080 ) ) ;
#22526=CIRCLE ( 'NONE', #4206, 5.000000000000000000 ) ;
#22529=CARTESIAN_POINT ( 'NONE',  ( 15.41947860041720908, 17.49999999999956302, 154.5727510624243166 ) ) ;
#22538=CARTESIAN_POINT ( 'NONE',  ( 0.2485248900955927820, 30.22197614145972366, 152.9047840822881881 ) ) ;
#22563=ORIENTED_EDGE ( 'NONE', *, *, #20756, .F. ) ;
#22575=AXIS2_PLACEMENT_3D ( 'NONE', #7656, #11664, #24663 ) ;
#22586=CARTESIAN_POINT ( 'NONE',  ( -16.28249153430137497, 8.099299129593275026, 159.5815388724490163 ) ) ;
#22666=ORIENTED_EDGE ( 'NONE', *, *, #13485, .T. ) ;
#22669=FACE_OUTER_BOUND ( 'NONE', #16971, .T. ) ;
#22672=ORIENTED_EDGE ( 'NONE', *, *, #35986, .F. ) ;
#22689=DIRECTION ( 'NONE',  ( -0.5000000000000038858, 0.8660254037844363761, 0.000000000000000000 ) ) ;
#22695=CARTESIAN_POINT ( 'NONE',  ( 11.28839907014777211, 11.57474747238952162, 152.9200731080177889 ) ) ;
#22712=CARTESIAN_POINT ( 'NONE',  ( -9.722444945199821831, 28.68682341637555311, 154.2021328665915405 ) ) ;
#22726=CARTESIAN_POINT ( 'NONE',  ( 13.03350328710527073, 15.16811627926489159, 153.2251063045275998 ) ) ;
#22734=CARTESIAN_POINT ( 'NONE',  ( 10.20684115509065926, 26.69374788516359942, 153.5324451153148573 ) ) ;
#22744=DIRECTION ( 'NONE',  ( 0.000000000000000000, 0.000000000000000000, -1.000000000000000000 ) ) ;
#22745=ADVANCED_FACE ( 'NONE', ( #17970 ), #27125, .F. ) ;
#22751=DIRECTION ( 'NONE',  ( -0.000000000000000000, -0.000000000000000000, 1.000000000000000000 ) ) ;
#22756=CARTESIAN_POINT ( 'NONE',  ( -1.987944452395423278, 30.53474097353426586, 153.1863241160601490 ) ) ;
#22771=B_SPLINE_CURVE_WITH_KNOTS ( 'NONE', 3,
 ( #34945, #11762, #15601, #27727, #41547, #28559, #25388, #5813, #40696, #18787, #12400, #24544, #5184, #14966, #37511, #38347, #8366, #6849, #16437, #12613, #19608, #29386, #6644, #16032, #25595, #12819 ),
 .UNSPECIFIED., .F., .F.,
 ( 4, 2, 2, 2, 2, 2, 2, 2, 2, 2, 2, 2, 4 ),
 ( 2.406822060230895526E-07, 0.001294128252029592150, 0.001941072036941364314, 0.002588015821853136261, 0.003234959606764908641, 0.003881903391676680588, 0.005175790961500214074, 0.006469678531323751029, 0.007116622316235519073, 0.007763566101147287117, 0.008410509886059056028, 0.009057453670970824072, 0.01035134124079433587 ),
 .UNSPECIFIED. ) ;
#22823=CARTESIAN_POINT ( 'NONE',  ( -5.209739300209230706, 8.476466837849001124, 159.5815388724490163 ) ) ;
#22825=DIRECTION ( 'NONE',  ( -0.8660254037844397068, 0.4999999999999979461, 0.000000000000000000 ) ) ;
#22826=VECTOR ( 'NONE', #2056, 1000.000000000000000 ) ;
#22850=CARTESIAN_POINT ( 'NONE',  ( -8.901842255144094551, 9.850514164664668115, 152.2937014009054906 ) ) ;
#22891=DIRECTION ( 'NONE',  ( 0.8505458157821428333, 0.000000000000000000, 0.5259009557468868890 ) ) ;
#22895=DIRECTION ( 'NONE',  ( -1.000000000000000000, 0.000000000000000000, 0.000000000000000000 ) ) ;
#22926=ORIENTED_EDGE ( 'NONE', *, *, #39109, .T. ) ;
#23001=FACE_OUTER_BOUND ( 'NONE', #30208, .T. ) ;
#23076=VERTEX_POINT ( 'NONE', #6249 ) ;
#23091=EDGE_CURVE ( 'NONE', #31801, #37892, #25823, .T. ) ;
#23096=CARTESIAN_POINT ( 'NONE',  ( 2.858598646995991643, 4.063742324715648557, 159.5815388724490163 ) ) ;
#23097=DIRECTION ( 'NONE',  ( 0.000000000000000000, 0.000000000000000000, -1.000000000000000000 ) ) ;
#23102=DIRECTION ( 'NONE',  ( -0.8660254037844363761, -0.5000000000000038858, 0.000000000000000000 ) ) ;
#23105=EDGE_CURVE ( 'NONE', #30300, #36157, #6663, .T. ) ;
#23172=CARTESIAN_POINT ( 'NONE',  ( 0.5068703235616166536, 30.23811901112014411, 152.9195735263550660 ) ) ;
#23186=CARTESIAN_POINT ( 'NONE',  ( -15.19684507887559910, 18.99101325121422690, 154.4793021320813864 ) ) ;
#23188=ORIENTED_EDGE ( 'NONE', *, *, #30520, .F. ) ;
#23199=CARTESIAN_POINT ( 'NONE',  ( -1.000000000000119460, 28.78848757896615496, 154.5815388724490163 ) ) ;
#23203=CARTESIAN_POINT ( 'NONE',  ( 0.000000000000000000, 0.000000000000000000, 154.5815388724490163 ) ) ;
#23210=CYLINDRICAL_SURFACE ( 'NONE', #7721, 3.499999999999999556 ) ;
#23214=CARTESIAN_POINT ( 'NONE',  ( -9.416638889553262004, 5.766054133116472968, 154.3405383956092578 ) ) ;
#23219=EDGE_CURVE ( 'NONE', #19996, #23076, #10275, .T. ) ;
#23245=DIRECTION ( 'NONE',  ( -0.000000000000000000, -0.000000000000000000, -1.000000000000000000 ) ) ;
#23276=VECTOR ( 'NONE', #13422, 1000.000000000000000 ) ;
#23282=CARTESIAN_POINT ( 'NONE',  ( -13.30584406242307871, 15.51494676818789031, 153.3565333127149302 ) ) ;
#23292=PLANE ( 'NONE',  #21907 ) ;
#23309=B_SPLINE_CURVE_WITH_KNOTS ( 'NONE', 3,
 ( #39693, #139, #7163, #6536, #35868, #22695, #35673, #16532, #9946, #19502, #29698, #33094, #26519, #29909, #3961, #16325 ),
 .UNSPECIFIED., .F., .F.,
 ( 4, 2, 2, 2, 2, 2, 2, 4 ),
 ( 2.508354784725399838E-07, 0.001523425935721374859, 0.002285013485842833213, 0.003046601035964291351, 0.003808188586085749922, 0.004569776136207207191, 0.005331363686328665329, 0.006092951236450123466 ),
 .UNSPECIFIED. ) ;
#23317=DIRECTION ( 'NONE',  ( 1.000000000000000000, 0.000000000000000000, 0.000000000000000000 ) ) ;
#23322=DIRECTION ( 'NONE',  ( 1.000000000000000000, 0.000000000000000000, 0.000000000000000000 ) ) ;
#23328=CARTESIAN_POINT ( 'NONE',  ( 15.36329688951068917, 18.36329766863108048, 154.5493626814884749 ) ) ;
#23353=CARTESIAN_POINT ( 'NONE',  ( -8.153942370607127899, 28.42187071401897924, 153.4658061086806811 ) ) ;
#23372=APPLICATION_CONTEXT ( 'automotive_design' ) ;
#23382=PLANE ( 'NONE',  #30431 ) ;
#23411=VECTOR ( 'NONE', #2603, 1000.000000000000000 ) ;
#23433=EDGE_CURVE ( 'NONE', #6544, #14462, #3377, .T. ) ;
#23460=ADVANCED_FACE ( 'NONE', ( #35918 ), #29538, .T. ) ;
#23462=DIRECTION ( 'NONE',  ( 0.000000000000000000, 0.000000000000000000, 1.000000000000000000 ) ) ;
#23464=AXIS2_PLACEMENT_3D ( 'NONE', #4225, #3800, #36121 ) ;
#23526=ADVANCED_FACE ( 'NONE', ( #30389 ), #36776, .T. ) ;
#23542=CYLINDRICAL_SURFACE ( 'NONE', #313, 6.079174044924941178 ) ;
#23564=DIRECTION ( 'NONE',  ( 0.4999999999999919509, 0.8660254037844432595, 0.000000000000000000 ) ) ;
#23599=CARTESIAN_POINT ( 'NONE',  ( -10.41947860041774199, 17.49999999999951683, 159.5815388724490163 ) ) ;
#23603=PLANE ( 'NONE',  #33483 ) ;
#23640=CARTESIAN_POINT ( 'NONE',  ( 2.858598646995926362, 30.93625767528271098, 150.5815388724490163 ) ) ;
#23648=CARTESIAN_POINT ( 'NONE',  ( 9.067620284531816566, 10.44167617710908402, 152.1415020426163665 ) ) ;
#23657=CARTESIAN_POINT ( 'NONE',  ( -2.858598646996156400, 4.063742324715559739, 153.5324451153154541 ) ) ;
#23663=CARTESIAN_POINT ( 'NONE',  ( 11.30060084420212974, 21.15496178874873223, 152.3738872609092994 ) ) ;
#23671=CARTESIAN_POINT ( 'NONE',  ( 12.28618350919697200, 22.31318234678377266, 153.1965160676642199 ) ) ;
#23735=FACE_OUTER_BOUND ( 'NONE', #33001, .T. ) ;
#23769=AXIS2_PLACEMENT_3D ( 'NONE', #5905, #21643, #2081 ) ;
#23793=ADVANCED_FACE ( 'NONE', ( #25691 ), #5699, .F. ) ;
#23824=AXIS2_PLACEMENT_3D ( 'NONE', #16687, #29428, #299 ) ;
#23830=CARTESIAN_POINT ( 'NONE',  ( -4.742640687119331844, 19.08346433899860273, 154.5815388724490163 ) ) ;
#23843=ADVANCED_FACE ( 'NONE', ( #15279 ), #15490, .F. ) ;
#23858=CARTESIAN_POINT ( 'NONE',  ( 2.858598646995926362, 30.93625767528271098, 153.5324451153149141 ) ) ;
#23871=CARTESIAN_POINT ( 'NONE',  ( -10.19301642060158741, 7.900390593925620486, 153.6940459180249263 ) ) ;
#23877=CARTESIAN_POINT ( 'NONE',  ( 4.935610658065304079, 30.01587512093893650, 153.3570253102923573 ) ) ;
#23890=ORIENTED_EDGE ( 'NONE', *, *, #18414, .F. ) ;
#23892=CARTESIAN_POINT ( 'NONE',  ( -10.20684115509089906, 26.69374788516367403, 153.5324451153149994 ) ) ;
#23895=EDGE_CURVE ( 'NONE', #23076, #32078, #17770, .T. ) ;
#23911=CARTESIAN_POINT ( 'NONE',  ( 13.41035298162382539, 13.47260506786468248, 153.6942049793718468 ) ) ;
#23928=CARTESIAN_POINT ( 'NONE',  ( 1.012168522246104541, 4.698199547958351374, 152.9774433921730292 ) ) ;
#23934=AXIS2_PLACEMENT_3D ( 'NONE', #10004, #40399, #30407 ) ;
#23944=EDGE_CURVE ( 'NONE', #36248, #18842, #10852, .T. ) ;
#23947=CARTESIAN_POINT ( 'NONE',  ( 15.41947860041720553, 17.49999999999956302, 159.5815388724490163 ) ) ;
#23961=AXIS2_PLACEMENT_3D ( 'NONE', #12381, #38120, #27916 ) ;
#23989=ORIENTED_EDGE ( 'NONE', *, *, #24857, .T. ) ;
#24001=CIRCLE ( 'NONE', #39569, 5.000000000000000000 ) ;
#24003=CARTESIAN_POINT ( 'NONE',  ( -14.96450702994103743, 19.59493642599608876, 154.3807879069782700 ) ) ;
#24027=CARTESIAN_POINT ( 'NONE',  ( -2.604869650104253420, 31.41246745148119857, 159.5815388724490163 ) ) ;
#24036=CIRCLE ( 'NONE', #5676, 7.579174044925158782 ) ;
#24044=EDGE_CURVE ( 'NONE', #24301, #14462, #30451, .T. ) ;
#24049=DIRECTION ( 'NONE',  ( 0.000000000000000000, 0.000000000000000000, -1.000000000000000000 ) ) ;
#24050=AXIS2_PLACEMENT_3D ( 'NONE', #1523, #1315, #8726 ) ;
#24059=ADVANCED_FACE ( 'NONE', ( #10680 ), #40023, .T. ) ;
#24097=VECTOR ( 'NONE', #42061, 999.9999999999998863 ) ;
#24102=CARTESIAN_POINT ( 'NONE',  ( -11.14833699762147390, 23.63548457597488550, 152.9052493666960402 ) ) ;
#24112=DIRECTION ( 'NONE',  ( 0.000000000000000000, 0.000000000000000000, 1.000000000000000000 ) ) ;
#24128=EDGE_CURVE ( 'NONE', #20998, #1168, #7702, .T. ) ;
#24135=EDGE_LOOP ( 'NONE', ( #34521, #29656, #37721 ) ) ;
#24144=CARTESIAN_POINT ( 'NONE',  ( 3.563940842959631539, 29.61244032134256088, 152.8454421597755299 ) ) ;
#24148=EDGE_LOOP ( 'NONE', ( #38150, #24619, #3607, #11349 ) ) ;
#24151=ORIENTED_EDGE ( 'NONE', *, *, #32346, .T. ) ;
#24160=DIRECTION ( 'NONE',  ( -1.000000000000000000, 0.000000000000000000, 0.000000000000000000 ) ) ;
#24186=ORIENTED_EDGE ( 'NONE', *, *, #41102, .T. ) ;
#24233=CARTESIAN_POINT ( 'NONE',  ( 13.91947860041720908, 17.49999999999956302, 153.6452861111154675 ) ) ;
#24242=ORIENTED_EDGE ( 'NONE', *, *, #2956, .F. ) ;
#24262=CARTESIAN_POINT ( 'NONE',  ( 5.209739300208925172, 8.476466837849169877, 159.5815388724490163 ) ) ;
#24265=DIRECTION ( 'NONE',  ( -0.000000000000000000, -0.000000000000000000, -1.000000000000000000 ) ) ;
#24272=CARTESIAN_POINT ( 'NONE',  ( 12.02068193548561581, 14.37371891743976171, 152.7173827546449161 ) ) ;
#24298=CARTESIAN_POINT ( 'NONE',  ( 9.718734271692362370, 11.88888615205622123, 159.5815388724490163 ) ) ;
#24301=VERTEX_POINT ( 'NONE', #28295 ) ;
#24332=DIRECTION ( 'NONE',  ( 0.8660254037844328234, 0.5000000000000101030, 0.000000000000000000 ) ) ;
#24340=FACE_OUTER_BOUND ( 'NONE', #40412, .T. ) ;
#24344=CARTESIAN_POINT ( 'NONE',  ( -10.03587323178440194, 23.29421411192350178, 159.5815388724490163 ) ) ;
#24345=AXIS2_PLACEMENT_3D ( 'NONE', #23599, #14025, #33589 ) ;
#24429=DIRECTION ( 'NONE',  ( 0.000000000000000000, 0.000000000000000000, -1.000000000000000000 ) ) ;
#24439=DIRECTION ( 'NONE',  ( 0.000000000000000000, 0.000000000000000000, -1.000000000000000000 ) ) ;
#24458=EDGE_LOOP ( 'NONE', ( #24186, #14618, #14737, #12676, #32058, #24705 ) ) ;
#24474=CIRCLE ( 'NONE', #30577, 5.000000000000004441 ) ;
#24479=CARTESIAN_POINT ( 'NONE',  ( 12.27165144158615284, 14.53024314691610641, 152.8454421597757289 ) ) ;
#24490=FACE_OUTER_BOUND ( 'NONE', #13308, .T. ) ;
#24494=AXIS2_PLACEMENT_3D ( 'NONE', #31815, #12472, #37580 ) ;
#24513=LINE ( 'NONE', #8546, #39738 ) ;
#24533=CARTESIAN_POINT ( 'NONE',  ( -16.28249153430137852, 26.90070087040669478, 159.5815388724490163 ) ) ;
#24544=CARTESIAN_POINT ( 'NONE',  ( 6.926659451089854258, 3.760829132662153018, 154.5487360771612941 ) ) ;
#24549=CARTESIAN_POINT ( 'NONE',  ( -1.254681948488981735, 4.652094401957341141, 153.0192156368757992 ) ) ;
#24561=EDGE_CURVE ( 'NONE', #35681, #41665, #15580, .T. ) ;
#24619=ORIENTED_EDGE ( 'NONE', *, *, #29359, .T. ) ;
#24632=DIRECTION ( 'NONE',  ( -1.000000000000000000, 0.000000000000000000, 0.000000000000000000 ) ) ;
#24650=EDGE_CURVE ( 'NONE', #5552, #37842, #21655, .T. ) ;
#24651=CYLINDRICAL_SURFACE ( 'NONE', #28768, 6.079174044926197951 ) ;
#24663=DIRECTION ( 'NONE',  ( -1.000000000000000000, 0.000000000000000000, 0.000000000000000000 ) ) ;
#24665=ORIENTED_EDGE ( 'NONE', *, *, #16512, .F. ) ;
#24682=VECTOR ( 'NONE', #1197, 1000.000000000000000 ) ;
#24705=ORIENTED_EDGE ( 'NONE', *, *, #29319, .T. ) ;
#24711=ORIENTED_EDGE ( 'NONE', *, *, #15741, .T. ) ;
#24712=CARTESIAN_POINT ( 'NONE',  ( 0.000000000000000000, 36.30140174081339666, 154.5815388724490163 ) ) ;
#24720=ORIENTED_EDGE ( 'NONE', *, *, #712, .T. ) ;
#24724=CIRCLE ( 'NONE', #13151, 5.000000000000004441 ) ;
#24725=ORIENTED_EDGE ( 'NONE', *, *, #9232, .T. ) ;
#24751=CARTESIAN_POINT ( 'NONE',  ( 10.41947860041720375, 17.49999999999957012, 159.5815388724490163 ) ) ;
#24766=ORIENTED_EDGE ( 'NONE', *, *, #160, .F. ) ;
#24787=CARTESIAN_POINT ( 'NONE',  ( -3.563940842960078292, 5.387559678655591711, 159.5815388724490163 ) ) ;
#24818=EDGE_LOOP ( 'NONE', ( #361, #10687, #19779, #7767 ) ) ;
#24820=VECTOR ( 'NONE', #28593, 1000.000000000000000 ) ;
#24828=CARTESIAN_POINT ( 'NONE',  ( 5.209739300208269697, 26.52353316214887613, 159.5815388724490163 ) ) ;
#24829=CARTESIAN_POINT ( 'NONE',  ( -10.41947860041774199, 17.49999999999951683, 159.5815388724490163 ) ) ;
#24853=CARTESIAN_POINT ( 'NONE',  ( 8.707710598626619003, 8.357316531739469312, 152.8454421597759847 ) ) ;
#24857=EDGE_CURVE ( 'NONE', #32078, #10573, #4585, .T. ) ;
#24866=CARTESIAN_POINT ( 'NONE',  ( 3.563940842959631539, 29.61244032134256088, 152.8454421597755299 ) ) ;
#24869=CARTESIAN_POINT ( 'NONE',  ( -2.485010488553506036, 5.885911749694646922, 152.3738872082082878 ) ) ;
#24877=EDGE_CURVE ( 'NONE', #1899, #645, #4556, .T. ) ;
#24879=DIRECTION ( 'NONE',  ( 0.000000000000000000, 0.000000000000000000, -1.000000000000000000 ) ) ;
#24894=CARTESIAN_POINT ( 'NONE',  ( 7.222421200248660966, 5.596585881668000972, 153.6454670892167371 ) ) ;
#24899=AXIS2_PLACEMENT_3D ( 'NONE', #34853, #28258, #2101 ) ;
#24912=LINE ( 'NONE', #15125, #34228 ) ;
#24921=ORIENTED_EDGE ( 'NONE', *, *, #31697, .T. ) ;
#24964=DIRECTION ( 'NONE',  ( -0.8825449026267668806, -0.4702281306424686558, -0.000000000000000000 ) ) ;
#24992=CARTESIAN_POINT ( 'NONE',  ( 2.858598646995927695, 30.93625767528271453, 159.5815388724490163 ) ) ;
#25031=VECTOR ( 'NONE', #8946, 1000.000000000000000 ) ;
#25036=ORIENTED_EDGE ( 'NONE', *, *, #1785, .T. ) ;
#25058=AXIS2_PLACEMENT_3D ( 'NONE', #3577, #32091, #25933 ) ;
#25088=CIRCLE ( 'NONE', #37992, 4.999999999999999112 ) ;
#25100=CARTESIAN_POINT ( 'NONE',  ( 3.812946306956437326, 5.254887252010445486, 152.9675983386013911 ) ) ;
#25125=LINE ( 'NONE', #8738, #4152 ) ;
#25136=EDGE_CURVE ( 'NONE', #16759, #33258, #13535, .T. ) ;
#25155=DIRECTION ( 'NONE',  ( 0.000000000000000000, 0.000000000000000000, 1.000000000000000000 ) ) ;
#25185=EDGE_LOOP ( 'NONE', ( #34478, #28620, #20100, #15031 ) ) ;
#25218=ORIENTED_EDGE ( 'NONE', *, *, #32189, .T. ) ;
#25236=DIRECTION ( 'NONE',  ( 0.9994203709764779564, 0.03404294460294525482, 0.000000000000000000 ) ) ;
#25254=FACE_OUTER_BOUND ( 'NONE', #37420, .T. ) ;
#25354=CIRCLE ( 'NONE', #4973, 11.07917404492494029 ) ;
#25373=EDGE_LOOP ( 'NONE', ( #38673, #31703, #19301, #3361, #36413, #8464, #41287, #8883 ) ) ;
#25386=AXIS2_PLACEMENT_3D ( 'NONE', #41328, #6433, #15808 ) ;
#25388=CARTESIAN_POINT ( 'NONE',  ( 5.032437754690803899, 3.475176470060715062, 154.2509714831756469 ) ) ;
#25401=DIRECTION ( 'NONE',  ( 1.000000000000000000, 0.000000000000000000, 0.000000000000000000 ) ) ;
#25435=EDGE_CURVE ( 'NONE', #21263, #20517, #34606, .T. ) ;
#25454=CARTESIAN_POINT ( 'NONE',  ( -8.707710598626180243, 26.64268346825927836, 159.5815388724490163 ) ) ;
#25456=CYLINDRICAL_SURFACE ( 'NONE', #24494, 4.999999999999999112 ) ;
#25459=CARTESIAN_POINT ( 'NONE',  ( -15.41947860041774376, 17.49999999999956657, 154.5727510624246293 ) ) ;
#25472=CARTESIAN_POINT ( 'NONE',  ( -10.43622283668263506, 22.06694147210445678, 152.0797566693945555 ) ) ;
#25474=FACE_OUTER_BOUND ( 'NONE', #13880, .T. ) ;
#25479=CARTESIAN_POINT ( 'NONE',  ( 0.000000000000000000, 17.49999999999998934, 141.5815388724490163 ) ) ;
#25484=DIRECTION ( 'NONE',  ( 1.000000000000000000, -0.000000000000000000, 0.000000000000000000 ) ) ;
#25498=CARTESIAN_POINT ( 'NONE',  ( -5.827333669639131131, 5.028125020260302058, 153.5499869721893162 ) ) ;
#25499=ORIENTED_EDGE ( 'NONE', *, *, #11348, .F. ) ;
#25500=CARTESIAN_POINT ( 'NONE',  ( -5.819810511207727188, 29.97322724569556840, 153.5487751394672671 ) ) ;
#25522=B_SPLINE_CURVE_WITH_KNOTS ( 'NONE', 3,
 ( #6831, #20236, #39802, #23648, #35768, #20449, #39155, #32565, #33415, #36, #3432, #26207, #21484, #5112, #24272, #24479 ),
 .UNSPECIFIED., .F., .F.,
 ( 4, 2, 2, 2, 2, 2, 2, 4 ),
 ( 2.157098444381531571E-07, 0.001910958079630934369, 0.002866329264524179396, 0.003821700449417424639, 0.004777071634310669015, 0.005732442819203913825, 0.006687814004097158635, 0.007643185188990402577 ),
 .UNSPECIFIED. ) ;
#25537=ORIENTED_EDGE ( 'NONE', *, *, #22299, .F. ) ;
#25561=EDGE_LOOP ( 'NONE', ( #4035, #32295, #919 ) ) ;
#25595=CARTESIAN_POINT ( 'NONE',  ( 10.19301004761593532, 7.900203498142930769, 153.6941204134551811 ) ) ;
#25606=DIRECTION ( 'NONE',  ( -0.03404294460276021533, 0.9994203709764843957, -0.000000000000000000 ) ) ;
#25635=CARTESIAN_POINT ( 'NONE',  ( -11.30060084420261646, 13.84503821125029965, 152.3738872609096404 ) ) ;
#25661=DIRECTION ( 'NONE',  ( -1.000000000000000000, 0.000000000000000000, 0.000000000000000000 ) ) ;
#25663=DIRECTION ( 'NONE',  ( -0.8660254037844397068, 0.4999999999999979461, 0.000000000000000000 ) ) ;
#25691=FACE_OUTER_BOUND ( 'NONE', #38308, .T. ) ;
#25702=CARTESIAN_POINT ( 'NONE',  ( -3.216997096249671895, 31.12721570168584861, 153.6940457802674018 ) ) ;
#25706=CARTESIAN_POINT ( 'NONE',  ( -8.487683822072755291, 7.240888989248395191, 153.2711608817841409 ) ) ;
#25723=CARTESIAN_POINT ( 'NONE',  ( 6.312108301366492924, 31.40528732289386227, 154.4799523715088867 ) ) ;
#25739=CARTESIAN_POINT ( 'NONE',  ( 16.28249153430137852, 26.90070087040669122, 159.5815388724490163 ) ) ;
#25749=ORIENTED_EDGE ( 'NONE', *, *, #37103, .T. ) ;
#25780=CARTESIAN_POINT ( 'NONE',  ( -1.196959198423996895E-13, 29.08842822384727356, 154.5815388724490163 ) ) ;
#25803=CARTESIAN_POINT ( 'NONE',  ( -1.196959198423996895E-13, 28.72222769588706015, 154.5815388724490163 ) ) ;
#25811=CARTESIAN_POINT ( 'NONE',  ( 9.718734271691504389, 23.11111384794381252, 159.5815388724490163 ) ) ;
#25823=LINE ( 'NONE', #28992, #5409 ) ;
#25842=CARTESIAN_POINT ( 'NONE',  ( -12.27165144158654542, 14.53024314691596963, 152.8454421597759563 ) ) ;
#25893=CARTESIAN_POINT ( 'NONE',  ( 15.12794563354680655, 19.19585752040785920, 154.4502191185280253 ) ) ;
#25894=CARTESIAN_POINT ( 'NONE',  ( -13.87922053742563300, 18.10975912486529182, 153.6267098343902262 ) ) ;
#25911=CARTESIAN_POINT ( 'NONE',  ( -8.426051298354920505, 30.37610395949893416, 154.5496813259655084 ) ) ;
#25916=CARTESIAN_POINT ( 'NONE',  ( -4.082076315226684571, 5.150617007611492326, 153.0794453411715494 ) ) ;
#25933=DIRECTION ( 'NONE',  ( -1.000000000000000000, 0.000000000000000000, 0.000000000000000000 ) ) ;
#25966=AXIS2_PLACEMENT_3D ( 'NONE', #19203, #35782, #28761 ) ;
#26020=AXIS2_PLACEMENT_3D ( 'NONE', #29774, #24049, #20846 ) ;
#26049=AXIS2_PLACEMENT_3D ( 'NONE', #33522, #20334, #23322 ) ;
#26060=AXIS2_PLACEMENT_3D ( 'NONE', #7643, #4862, #1878 ) ;
#26069=SHAPE_DEFINITION_REPRESENTATION ( #33989, #19321 ) ;
#26081=ORIENTED_EDGE ( 'NONE', *, *, #23433, .F. ) ;
#26093=DIRECTION ( 'NONE',  ( -0.000000000000000000, -0.000000000000000000, 1.000000000000000000 ) ) ;
#26130=VECTOR ( 'NONE', #3338, 1000.000000000000000 ) ;
#26146=AXIS2_PLACEMENT_3D ( 'NONE', #34402, #12486, #24632 ) ;
#26168=FACE_OUTER_BOUND ( 'NONE', #30760, .T. ) ;
#26175=CARTESIAN_POINT ( 'NONE',  ( 4.330127018922108384, 20.00000000000014211, 154.5815388724490163 ) ) ;
#26207=CARTESIAN_POINT ( 'NONE',  ( 11.07557039803270982, 13.61552157711410516, 152.2937014864025684 ) ) ;
#26208=AXIS2_PLACEMENT_3D ( 'NONE', #1771, #5170, #18143 ) ;
#26218=ORIENTED_EDGE ( 'NONE', *, *, #6896, .F. ) ;
#26227=CARTESIAN_POINT ( 'NONE',  ( 13.06543980208692091, 21.74250979011892326, 153.5324451153149710 ) ) ;
#26237=AXIS2_PLACEMENT_3D ( 'NONE', #38936, #22348, #13196 ) ;
#26239=ADVANCED_FACE ( 'NONE', ( #40694 ), #37509, .T. ) ;
#26283=ORIENTED_EDGE ( 'NONE', *, *, #1277, .T. ) ;
#26313=CARTESIAN_POINT ( 'NONE',  ( 13.73174959043948817, 21.26813471983483339, 153.8403160775951619 ) ) ;
#26330=CARTESIAN_POINT ( 'NONE',  ( -8.083882785675909233, 30.63816656191788113, 154.5729385747524987 ) ) ;
#26350=CARTESIAN_POINT ( 'NONE',  ( 9.416638889552039871, 29.23394586688180752, 154.3405383956084052 ) ) ;
#26359=DIRECTION ( 'NONE',  ( -0.000000000000000000, -0.000000000000000000, 1.000000000000000000 ) ) ;
#26360=DIRECTION ( 'NONE',  ( -1.000000000000000000, 0.000000000000000000, 0.000000000000000000 ) ) ;
#26371=DIRECTION ( 'NONE',  ( 0.000000000000000000, 1.000000000000000000, 0.000000000000000000 ) ) ;
#26384=VECTOR ( 'NONE', #41286, 1000.000000000000000 ) ;
#26392=VERTEX_POINT ( 'NONE', #32173 ) ;
#26469=ORIENTED_EDGE ( 'NONE', *, *, #34771, .F. ) ;
#26479=CIRCLE ( 'NONE', #19004, 5.000000000000004441 ) ;
#26480=EDGE_CURVE ( 'NONE', #28419, #27996, #35963, .T. ) ;
#26484=ORIENTED_EDGE ( 'NONE', *, *, #39731, .T. ) ;
#26519=CARTESIAN_POINT ( 'NONE',  ( 10.31142999045256836, 9.266444396987289167, 153.1965159924009185 ) ) ;
#26539=DIRECTION ( 'NONE',  ( 0.000000000000000000, 0.000000000000000000, -1.000000000000000000 ) ) ;
#26549=AXIS2_PLACEMENT_3D ( 'NONE', #32225, #14021, #11035 ) ;
#26560=CARTESIAN_POINT ( 'NONE',  ( 9.629634397220087294, 28.87063105448513767, 154.2509715743847210 ) ) ;
#26591=EDGE_LOOP ( 'NONE', ( #3772, #27224, #41034, #20432, #36312, #19819, #27060, #29295 ) ) ;
#26629=ORIENTED_EDGE ( 'NONE', *, *, #14001, .T. ) ;
#26631=CARTESIAN_POINT ( 'NONE',  ( 5.084889071860446030, 30.02445155319908920, 153.3961973379644803 ) ) ;
#26666=EDGE_CURVE ( 'NONE', #8168, #21985, #26479, .T. ) ;
#26696=VERTEX_POINT ( 'NONE', #24853 ) ;
#26753=ORIENTED_EDGE ( 'NONE', *, *, #23895, .T. ) ;
#26765=EDGE_CURVE ( 'NONE', #31801, #29598, #23309, .T. ) ;
#26776=AXIS2_PLACEMENT_3D ( 'NONE', #34675, #37200, #30810 ) ;
#26804=CARTESIAN_POINT ( 'NONE',  ( 0.000000000000000000, 36.30140174081339666, 159.5815388724490163 ) ) ;
#26819=ORIENTED_EDGE ( 'NONE', *, *, #30262, .F. ) ;
#26826=PLANE ( 'NONE',  #29298 ) ;
#26869=AXIS2_PLACEMENT_3D ( 'NONE', #13805, #38123, #9620 ) ;
#26881=EDGE_CURVE ( 'NONE', #10531, #20414, #29853, .T. ) ;
#26888=CARTESIAN_POINT ( 'NONE',  ( -11.59049936059954611, 11.97299561512788202, 152.9768715818108262 ) ) ;
#26904=VECTOR ( 'NONE', #36974, 1000.000000000000000 ) ;
#26911=VERTEX_POINT ( 'NONE', #19920 ) ;
#26937=CYLINDRICAL_SURFACE ( 'NONE', #26049, 6.079174044925958142 ) ;
#27057=CARTESIAN_POINT ( 'NONE',  ( 8.836825633739591623, 25.45247773631193411, 152.3877645506820500 ) ) ;
#27060=ORIENTED_EDGE ( 'NONE', *, *, #36280, .F. ) ;
#27065=ORIENTED_EDGE ( 'NONE', *, *, #10854, .F. ) ;
#27071=CARTESIAN_POINT ( 'NONE',  ( 1.000000000000119460, 12.60102051443365134, 155.5815388724490163 ) ) ;
#27096=CARTESIAN_POINT ( 'NONE',  ( -11.75395375419353172, 12.16263380007240968, 153.0192156799703582 ) ) ;
#27109=CARTESIAN_POINT ( 'NONE',  ( -13.53450912783562110, 15.89733096609164598, 153.4652957816663275 ) ) ;
#27125=CYLINDRICAL_SURFACE ( 'NONE', #37994, 3.500000000000000000 ) ;
#27160=DIRECTION ( 'NONE',  ( 0.8660254037844363761, 0.5000000000000038858, 0.000000000000000000 ) ) ;
#27179=EDGE_CURVE ( 'NONE', #35160, #20191, #30540, .T. ) ;
#27193=PRODUCT ( 'Long Screw Plastic Knob - Handle', 'Long Screw Plastic Knob - Handle', '', ( #12674 ) ) ;
#27224=ORIENTED_EDGE ( 'NONE', *, *, #27392, .F. ) ;
#27249=CARTESIAN_POINT ( 'NONE',  ( -10.03587323178440194, 23.29421411192350178, 154.5815388724490163 ) ) ;
#27272=CARTESIAN_POINT ( 'NONE',  ( 4.501085982074025438, 29.95406310662465188, 153.2263580705393622 ) ) ;
#27276=CARTESIAN_POINT ( 'NONE',  ( 8.158171636102967028, 28.41521699698126824, 153.4640812521331270 ) ) ;
#27290=DIRECTION ( 'NONE',  ( 0.000000000000000000, -0.000000000000000000, -1.000000000000000000 ) ) ;
#27351=CIRCLE ( 'NONE', #33449, 5.000000000000004441 ) ;
#27356=TOROIDAL_SURFACE ( 'NONE', #21215, 11.07917404492619795, 5.000000000000000000 ) ;
#27377=VERTEX_POINT ( 'NONE', #33045 ) ;
#27380=ORIENTED_EDGE ( 'NONE', *, *, #15211, .T. ) ;
#27383=ORIENTED_EDGE ( 'NONE', *, *, #23091, .F. ) ;
#27391=EDGE_LOOP ( 'NONE', ( #8380, #28093, #30565, #21299 ) ) ;
#27392=EDGE_CURVE ( 'NONE', #37104, #33855, #506, .T. ) ;
#27393=CARTESIAN_POINT ( 'NONE',  ( -14.87145978460237039, 19.78567178956339845, 154.3410716200992852 ) ) ;
#27411=DIRECTION ( 'NONE',  ( -1.000000000000000000, 0.000000000000000000, 0.000000000000000000 ) ) ;
#27458=CARTESIAN_POINT ( 'NONE',  ( -3.500000000000003997, 17.49999999999998934, 155.5815388724490163 ) ) ;
#27466=DIRECTION ( 'NONE',  ( -0.4702281306425868945, -0.8825449026267039310, 0.000000000000000000 ) ) ;
#27476=CARTESIAN_POINT ( 'NONE',  ( 5.381645978141616382, 30.02245660435134766, 153.4658060357136833 ) ) ;
#27488=CARTESIAN_POINT ( 'NONE',  ( 1.000000000000119460, 5.911571776152701574, 154.5815388724490163 ) ) ;
#27531=EDGE_CURVE ( 'NONE', #21985, #13202, #24474, .T. ) ;
#27554=DIRECTION ( 'NONE',  ( -0.000000000000000000, -0.000000000000000000, -1.000000000000000000 ) ) ;
#27567=EDGE_CURVE ( 'NONE', #3157, #9177, #31929, .T. ) ;
#27589=CARTESIAN_POINT ( 'NONE',  ( 0.000000000000000000, 36.30140174081339666, 159.5815388724490163 ) ) ;
#27595=CARTESIAN_POINT ( 'NONE',  ( 16.28249153430138207, 8.099299129593287461, 150.5815388724490163 ) ) ;
#27599=CARTESIAN_POINT ( 'NONE',  ( -14.15884394889474684, 20.82564817546664315, 154.0308563845583194 ) ) ;
#27610=LINE ( 'NONE', #37393, #39024 ) ;
#27624=DIRECTION ( 'NONE',  ( -0.000000000000000000, -0.000000000000000000, 1.000000000000000000 ) ) ;
#27690=EDGE_CURVE ( 'NONE', #13719, #37842, #5460, .T. ) ;
#27727=CARTESIAN_POINT ( 'NONE',  ( 4.197921810176673318, 3.575556083819466213, 154.0304303761510596 ) ) ;
#27732=AXIS2_PLACEMENT_3D ( 'NONE', #29747, #610, #4013 ) ;
#27737=ORIENTED_EDGE ( 'NONE', *, *, #14951, .F. ) ;
#27742=ORIENTED_EDGE ( 'NONE', *, *, #841, .F. ) ;
#27745=FACE_OUTER_BOUND ( 'NONE', #18272, .T. ) ;
#27751=ADVANCED_FACE ( 'NONE', ( #7318 ), #11149, .F. ) ;
#27798=ORIENTED_EDGE ( 'NONE', *, *, #14283, .F. ) ;
#27799=B_SPLINE_CURVE_WITH_KNOTS ( 'NONE', 3,
 ( #22734, #19332, #9776, #16364, #41894, #6357, #26560, #26350, #10181, #19747, #12743, #15949, #22514, #19537, #3379, #25723, #16572, #32714, #29307, #10396, #32508, #35908, #2959, #601, #3794, #29526 ),
 .UNSPECIFIED., .F., .F.,
 ( 4, 2, 2, 2, 2, 2, 2, 2, 2, 2, 2, 2, 4 ),
 ( 2.125331784069143882E-07, 0.001294100106467785827, 0.001941043893112474319, 0.002587987679757163244, 0.003234931466401851519, 0.003881875253046540662, 0.005175762826335915910, 0.006469650399625288990, 0.007116594186269977265, 0.007763537972914663805, 0.008410481759559350345, 0.009057425546204037753, 0.01035131311949343338 ),
 .UNSPECIFIED. ) ;
#27800=CARTESIAN_POINT ( 'NONE',  ( -14.66328716377165442, 20.15226711919136804, 154.2514967876348635 ) ) ;
#27811=CYLINDRICAL_SURFACE ( 'NONE', #26146, 3.500000000000003997 ) ;
#27860=CARTESIAN_POINT ( 'NONE',  ( 8.371260436320575593, 6.967698151607299550, 153.3570253316115668 ) ) ;
#27890=DIRECTION ( 'NONE',  ( 0.000000000000000000, 0.000000000000000000, 1.000000000000000000 ) ) ;
#27894=AXIS2_PLACEMENT_3D ( 'NONE', #35881, #14606, #27160 ) ;
#27907=AXIS2_PLACEMENT_3D ( 'NONE', #40090, #4363, #39879 ) ;
#27916=DIRECTION ( 'NONE',  ( 1.000000000000000000, 0.000000000000000000, 0.000000000000000000 ) ) ;
#27932=EDGE_CURVE ( 'NONE', #37892, #4470, #38773, .T. ) ;
#27970=LINE ( 'NONE', #5425, #40231 ) ;
#27978=ORIENTED_EDGE ( 'NONE', *, *, #10261, .F. ) ;
#27983=CIRCLE ( 'NONE', #6345, 7.579174044925481191 ) ;
#27989=VERTEX_POINT ( 'NONE', #40690 ) ;
#27996=VERTEX_POINT ( 'NONE', #28343 ) ;
#28019=CARTESIAN_POINT ( 'NONE',  ( 0.000000000000000000, 17.49999999999998934, 154.5815388724490163 ) ) ;
#28029=CARTESIAN_POINT ( 'NONE',  ( 8.707710598625942211, 26.64268346825921085, 152.8454421597755015 ) ) ;
#28041=EDGE_CURVE ( 'NONE', #18108, #2798, #11755, .T. ) ;
#28044=CARTESIAN_POINT ( 'NONE',  ( 16.28249153430137852, 26.90070087040669122, 159.5815388724490163 ) ) ;
#28047=ORIENTED_EDGE ( 'NONE', *, *, #18048, .T. ) ;
#28065=CARTESIAN_POINT ( 'NONE',  ( -5.000000000000004441, 17.49999999999998934, 141.5815388724490163 ) ) ;
#28069=CARTESIAN_POINT ( 'NONE',  ( 4.640808831584364746, 5.019894694007068559, 153.2711608748439573 ) ) ;
#28072=AXIS2_PLACEMENT_3D ( 'NONE', #25739, #22324, #35300 ) ;
#28084=ORIENTED_EDGE ( 'NONE', *, *, #40159, .F. ) ;
#28093=ORIENTED_EDGE ( 'NONE', *, *, #23219, .F. ) ;
#28163=VECTOR ( 'NONE', #30580, 1000.000000000000000 ) ;
#28208=DIRECTION ( 'NONE',  ( -0.000000000000000000, -0.000000000000000000, -1.000000000000000000 ) ) ;
#28217=EDGE_CURVE ( 'NONE', #18108, #9816, #12420, .T. ) ;
#28227=PLANE ( 'NONE',  #9163 ) ;
#28258=DIRECTION ( 'NONE',  ( 0.000000000000000000, 1.000000000000000000, 0.000000000000000000 ) ) ;
#28267=AXIS2_PLACEMENT_3D ( 'NONE', #17009, #26371, #7229 ) ;
#28295=CARTESIAN_POINT ( 'NONE',  ( 1.196959198423996895E-13, 6.277772304111523205, 154.5815388724490163 ) ) ;
#28327=CARTESIAN_POINT ( 'NONE',  ( 1.196959198423996895E-13, 6.277772304111523205, 159.5815388724490163 ) ) ;
#28336=ORIENTED_EDGE ( 'NONE', *, *, #11909, .T. ) ;
#28343=CARTESIAN_POINT ( 'NONE',  ( 3.500000000000003997, 17.49999999999998934, 141.5815388724490163 ) ) ;
#28350=FACE_OUTER_BOUND ( 'NONE', #35736, .T. ) ;
#28360=ORIENTED_EDGE ( 'NONE', *, *, #14951, .T. ) ;
#28419=VERTEX_POINT ( 'NONE', #31070 ) ;
#28434=CARTESIAN_POINT ( 'NONE',  ( 16.28249153430137852, 26.90070087040669122, 154.5815388724490163 ) ) ;
#28467=AXIS2_PLACEMENT_3D ( 'NONE', #26804, #14245, #29976 ) ;
#28523=VERTEX_POINT ( 'NONE', #8517 ) ;
#28525=DIRECTION ( 'NONE',  ( -1.000000000000000000, 0.000000000000000000, 0.000000000000000000 ) ) ;
#28559=CARTESIAN_POINT ( 'NONE',  ( 4.822789029776546776, 3.487033524486621960, 154.2011256547288269 ) ) ;
#28590=AXIS2_PLACEMENT_3D ( 'NONE', #14968, #40907, #21763 ) ;
#28593=DIRECTION ( 'NONE',  ( -0.000000000000000000, -0.000000000000000000, -1.000000000000000000 ) ) ;
#28620=ORIENTED_EDGE ( 'NONE', *, *, #13006, .T. ) ;
#28623=ORIENTED_EDGE ( 'NONE', *, *, #30520, .T. ) ;
#28643=DIRECTION ( 'NONE',  ( -0.000000000000000000, -0.000000000000000000, -1.000000000000000000 ) ) ;
#28644=CARTESIAN_POINT ( 'NONE',  ( -1.196959198423996895E-13, 28.72222769588706015, 159.5815388724490163 ) ) ;
#28667=CARTESIAN_POINT ( 'NONE',  ( -3.563940842959833599, 29.61244032134267101, 152.8454421597756152 ) ) ;
#28668=CARTESIAN_POINT ( 'NONE',  ( 1.570573766093340318, 6.119786567962919754, 152.1397377750291753 ) ) ;
#28676=DIRECTION ( 'NONE',  ( 0.000000000000000000, 0.000000000000000000, 1.000000000000000000 ) ) ;
#28692=CARTESIAN_POINT ( 'NONE',  ( 1.000000000000119460, 12.60102051443365134, 154.5815388724490163 ) ) ;
#28715=LINE ( 'NONE', #41499, #25031 ) ;
#28722=VERTEX_POINT ( 'NONE', #13766 ) ;
#28761=DIRECTION ( 'NONE',  ( -1.000000000000000000, 0.000000000000000000, 0.000000000000000000 ) ) ;
#28768=AXIS2_PLACEMENT_3D ( 'NONE', #37002, #7863, #31224 ) ;
#28770=ORIENTED_EDGE ( 'NONE', *, *, #9324, .T. ) ;
#28791=LINE ( 'NONE', #19439, #38111 ) ;
#28816=ADVANCED_FACE ( 'NONE', ( #9957 ), #13544, .F. ) ;
#28835=ORIENTED_EDGE ( 'NONE', *, *, #27179, .F. ) ;
#28836=CARTESIAN_POINT ( 'NONE',  ( -13.73174959044004062, 13.73186528016426422, 153.8403160775955030 ) ) ;
#28851=CARTESIAN_POINT ( 'NONE',  ( -10.64084095417646481, 21.82994978781176343, 152.1397378211945011 ) ) ;
#28864=CIRCLE ( 'NONE', #30238, 7.579174044926197062 ) ;
#28879=CARTESIAN_POINT ( 'NONE',  ( 0.3280984336919397504, 28.72259877500919245, 151.9779333920867828 ) ) ;
#28881=CARTESIAN_POINT ( 'NONE',  ( -7.887293579985452219, 28.78255665880528014, 153.5499870077382241 ) ) ;
#28903=CARTESIAN_POINT ( 'NONE',  ( 10.27611701369066743, 12.72178161430110066, 159.5815388724490163 ) ) ;
#28937=EDGE_LOOP ( 'NONE', ( #19422, #18754, #20644, #31085, #1672, #2955 ) ) ;
#28950=DIRECTION ( 'NONE',  ( 1.000000000000000000, 0.000000000000000000, 0.000000000000000000 ) ) ;
#28959=ORIENTED_EDGE ( 'NONE', *, *, #17565, .F. ) ;
#28969=ORIENTED_EDGE ( 'NONE', *, *, #41854, .F. ) ;
#28992=CARTESIAN_POINT ( 'NONE',  ( 13.06543980208709677, 13.25749020988032179, 150.5815388724490163 ) ) ;
#29041=CYLINDRICAL_SURFACE ( 'NONE', #4343, 3.500000000000001332 ) ;
#29056=CARTESIAN_POINT ( 'NONE',  ( 0.000000000000000000, 17.49999999999956302, 154.9135024962512546 ) ) ;
#29060=CARTESIAN_POINT ( 'NONE',  ( -12.27165144158644239, 20.46975685308312620, 152.8454421597758994 ) ) ;
#29084=CARTESIAN_POINT ( 'NONE',  ( -5.977173621346480559, 5.058257926121305204, 153.5727845806738117 ) ) ;
#29086=CARTESIAN_POINT ( 'NONE',  ( -5.373768961465406946, 30.02279240325918863, 153.4640811590190310 ) ) ;
#29125=VERTEX_POINT ( 'NONE', #34574 ) ;
#29144=ORIENTED_EDGE ( 'NONE', *, *, #19107, .T. ) ;
#29169=EDGE_LOOP ( 'NONE', ( #9763, #472, #8798, #9341, #11926 ) ) ;
#29213=CARTESIAN_POINT ( 'NONE',  ( -10.05866016940771956, 12.43597981122200657, 151.9992204325097305 ) ) ;
#29231=EDGE_CURVE ( 'NONE', #4470, #29783, #2754, .T. ) ;
#29237=FACE_OUTER_BOUND ( 'NONE', #34850, .T. ) ;
#29256=VECTOR ( 'NONE', #984, 1000.000000000000000 ) ;
#29268=CARTESIAN_POINT ( 'NONE',  ( -12.27165144158644239, 20.46975685308312620, 152.8454421597758994 ) ) ;
#29285=CARTESIAN_POINT ( 'NONE',  ( -9.957960250864815066, 28.10371618125153859, 154.0322826691235605 ) ) ;
#29287=AXIS2_PLACEMENT_3D ( 'NONE', #24712, #21508, #1534 ) ;
#29289=CARTESIAN_POINT ( 'NONE',  ( -7.892226332657691579, 6.223282550358369747, 153.5487751541058117 ) ) ;
#29291=CARTESIAN_POINT ( 'NONE',  ( -5.209739300209232482, 8.476466837849001124, 164.5815388724490163 ) ) ;
#29295=ORIENTED_EDGE ( 'NONE', *, *, #1751, .T. ) ;
#29296=VERTEX_POINT ( 'NONE', #8048 ) ;
#29298=AXIS2_PLACEMENT_3D ( 'NONE', #27249, #30002, #7892 ) ;
#29302=CARTESIAN_POINT ( 'NONE',  ( 13.71305093447463541, 16.30625799697444833, 153.5492497259775462 ) ) ;
#29307=CARTESIAN_POINT ( 'NONE',  ( 5.463316799720053574, 31.52158454959292655, 154.3424624008193291 ) ) ;
#29319=EDGE_CURVE ( 'NONE', #41665, #19996, #31330, .T. ) ;
#29340=ORIENTED_EDGE ( 'NONE', *, *, #5250, .T. ) ;
#29359=EDGE_CURVE ( 'NONE', #2094, #20998, #7113, .T. ) ;
#29366=CARTESIAN_POINT ( 'NONE',  ( 1.000000000000119460, 6.211512421032414188, 159.5815388724490163 ) ) ;
#29371=LINE ( 'NONE', #239, #23276 ) ;
#29386=CARTESIAN_POINT ( 'NONE',  ( 9.888348281643628113, 6.700247549245829326, 154.0918075026117435 ) ) ;
#29392=CARTESIAN_POINT ( 'NONE',  ( 10.88765427151083465, 24.08700026818530660, 152.9052493511307773 ) ) ;
#29398=ORIENTED_EDGE ( 'NONE', *, *, #7793, .T. ) ;
#29400=CARTESIAN_POINT ( 'NONE',  ( -4.330127018922262927, 19.99999999999987566, 159.5815388724490163 ) ) ;
#29428=DIRECTION ( 'NONE',  ( 0.000000000000000000, 0.000000000000000000, -1.000000000000000000 ) ) ;
#29435=AXIS2_PLACEMENT_3D ( 'NONE', #1516, #14704, #27466 ) ;
#29442=CARTESIAN_POINT ( 'NONE',  ( 12.27165144158600363, 20.46975685308311554, 159.5815388724490163 ) ) ;
#29453=ADVANCED_FACE ( 'NONE', ( #21972, #5815 ), #8794, .F. ) ;
#29458=ORIENTED_EDGE ( 'NONE', *, *, #34455, .F. ) ;
#29502=CARTESIAN_POINT ( 'NONE',  ( -15.15544456622774661, 26.24999999999984368, 154.5815388724490163 ) ) ;
#29508=CARTESIAN_POINT ( 'NONE',  ( -4.640808831584194216, 29.98010530599114887, 153.2711608748434458 ) ) ;
#29513=ADVANCED_FACE ( 'NONE', ( #24340 ), #8163, .T. ) ;
#29521=CARTESIAN_POINT ( 'NONE',  ( -5.209739300208508617, 26.52353316214900047, 159.5815388724490163 ) ) ;
#29525=VECTOR ( 'NONE', #11960, 1000.000000000000000 ) ;
#29526=CARTESIAN_POINT ( 'NONE',  ( 2.858598646995926362, 30.93625767528271098, 153.5324451153149141 ) ) ;
#29534=ADVANCED_FACE ( 'NONE', ( #17901 ), #22496, .T. ) ;
#29537=CARTESIAN_POINT ( 'NONE',  ( -16.28249153430137852, 26.90070087040669478, 159.5815388724490163 ) ) ;
#29538=CYLINDRICAL_SURFACE ( 'NONE', #31221, 4.999999999999999112 ) ;
#29551=ORIENTED_EDGE ( 'NONE', *, *, #38040, .T. ) ;
#29590=DIRECTION ( 'NONE',  ( -1.000000000000000000, 0.000000000000000000, 0.000000000000000000 ) ) ;
#29598=VERTEX_POINT ( 'NONE', #21510 ) ;
#29656=ORIENTED_EDGE ( 'NONE', *, *, #35265, .T. ) ;
#29679=CARTESIAN_POINT ( 'NONE',  ( 0.000000000000000000, 36.30140174081339666, 164.5815388724490163 ) ) ;
#29698=CARTESIAN_POINT ( 'NONE',  ( 10.49927174262173502, 9.989461018017575356, 153.0192155857725993 ) ) ;
#29699=CARTESIAN_POINT ( 'NONE',  ( -10.03587323178424562, 11.70578588807619091, 154.5815388724490163 ) ) ;
#29715=CARTESIAN_POINT ( 'NONE',  ( -10.19301004761542018, 27.09979650185599809, 153.6941204134548116 ) ) ;
#29747=CARTESIAN_POINT ( 'NONE',  ( 0.000000000000000000, 17.49999999999998934, 154.5815388724490163 ) ) ;
#29769=B_SPLINE_CURVE_WITH_KNOTS ( 'NONE', 3,
 ( #38359, #41142, #5400, #21775, #41560, #9009, #18377, #31348, #18798, #31141, #21987, #2212, #12414, #12199 ),
 .UNSPECIFIED., .F., .F.,
 ( 4, 2, 2, 2, 2, 2, 4 ),
 ( 0.003646029068602458199, 0.004555261728908127986, 0.005009878059060963312, 0.005464494389213797772, 0.005919110719366632231, 0.006373727049519467558, 0.007282959709825140814 ),
 .UNSPECIFIED. ) ;
#29774=CARTESIAN_POINT ( 'NONE',  ( -2.604869650104253420, 31.41246745148119857, 159.5815388724490163 ) ) ;
#29783=VERTEX_POINT ( 'NONE', #17905 ) ;
#29793=FACE_OUTER_BOUND ( 'NONE', #17704, .T. ) ;
#29805=CARTESIAN_POINT ( 'NONE',  ( -3.217162522966886318, 3.872696157419287744, 153.6941203706227839 ) ) ;
#29809=VECTOR ( 'NONE', #311, 1000.000000000000000 ) ;
#29828=CARTESIAN_POINT ( 'NONE',  ( -11.59276877416554186, 23.02433644519708622, 152.9774434186093686 ) ) ;
#29829=EDGE_CURVE ( 'NONE', #7502, #3564, #15033, .T. ) ;
#29847=CIRCLE ( 'NONE', #11510, 7.579174044925481191 ) ;
#29853=B_SPLINE_CURVE_WITH_KNOTS ( 'NONE', 3,
 ( #39478, #32676, #23328, #36289, #25893, #22477, #32885, #6319, #9735, #3750, #19294, #26313, #6944, #32269 ),
 .UNSPECIFIED., .F., .F.,
 ( 4, 2, 2, 2, 2, 2, 4 ),
 ( 0.005180900756485223857, 0.006473513313900679939, 0.007119819592608410581, 0.007766125871316142959, 0.008412432150023874469, 0.009058738428731605979, 0.01035135098614710022 ),
 .UNSPECIFIED. ) ;
#29856=CARTESIAN_POINT ( 'NONE',  ( -13.06543980208746092, 13.25749020988016547, 153.5324451153153120 ) ) ;
#29857=CARTESIAN_POINT ( 'NONE',  ( 0.000000000000000000, 17.49999999999998934, 154.5815388724490163 ) ) ;
#29874=EDGE_LOOP ( 'NONE', ( #30420, #23188, #37025, #20748 ) ) ;
#29880=DIRECTION ( 'NONE',  ( -0.5000000000000101030, 0.8660254037844328234, 0.000000000000000000 ) ) ;
#29905=CARTESIAN_POINT ( 'NONE',  ( -3.563940842960078292, 5.387559678655591711, 159.5815388724490163 ) ) ;
#29909=CARTESIAN_POINT ( 'NONE',  ( 10.23713785027279322, 8.784501924853445942, 153.3506917991490184 ) ) ;
#29937=ORIENTED_EDGE ( 'NONE', *, *, #37531, .T. ) ;
#29938=ORIENTED_EDGE ( 'NONE', *, *, #30448, .T. ) ;
#29953=CARTESIAN_POINT ( 'NONE',  ( -9.276117013690740265, 10.98973080673171765, 159.5815388724490163 ) ) ;
#29976=DIRECTION ( 'NONE',  ( -1.000000000000000000, 0.000000000000000000, 0.000000000000000000 ) ) ;
#29981=VERTEX_POINT ( 'NONE', #40651 ) ;
#29988=ORIENTED_EDGE ( 'NONE', *, *, #6193, .T. ) ;
#29992=ORIENTED_EDGE ( 'NONE', *, *, #10599, .T. ) ;
#30002=DIRECTION ( 'NONE',  ( -0.4999999999999980016, -0.8660254037844398178, 0.000000000000000000 ) ) ;
#30017=CARTESIAN_POINT ( 'NONE',  ( -9.629634397221311204, 6.129368945513225420, 154.2509715743855452 ) ) ;
#30025=EDGE_CURVE ( 'NONE', #9177, #1899, #25125, .T. ) ;
#30065=CARTESIAN_POINT ( 'NONE',  ( -10.77561899351985097, 10.68658643399665031, 152.9200730590040394 ) ) ;
#30136=DIRECTION ( 'NONE',  ( 1.000000000000000000, 0.000000000000000000, 0.000000000000000000 ) ) ;
#30147=EDGE_LOOP ( 'NONE', ( #11507, #15083, #10212, #24151, #2981, #2209 ) ) ;
#30149=DIRECTION ( 'NONE',  ( 0.000000000000000000, 0.000000000000000000, 1.000000000000000000 ) ) ;
#30153=EDGE_CURVE ( 'NONE', #8168, #2682, #28715, .T. ) ;
#30179=EDGE_LOOP ( 'NONE', ( #5801, #28360, #41809, #13824 ) ) ;
#30189=PLANE ( 'NONE',  #7620 ) ;
#30208=EDGE_LOOP ( 'NONE', ( #19000, #18474, #33210, #8752 ) ) ;
#30223=VECTOR ( 'NONE', #31672, 1000.000000000000000 ) ;
#30233=CARTESIAN_POINT ( 'NONE',  ( -6.312108301367226559, 3.594712677103959475, 154.4799523715097962 ) ) ;
#30238=AXIS2_PLACEMENT_3D ( 'NONE', #5778, #18755, #28525 ) ;
#30242=AXIS2_PLACEMENT_3D ( 'NONE', #6935, #10133, #22895 ) ;
#30258=DIRECTION ( 'NONE',  ( -0.8660254037844328234, -0.5000000000000101030, 0.000000000000000000 ) ) ;
#30262=EDGE_CURVE ( 'NONE', #6127, #40091, #5764, .T. ) ;
#30280=CARTESIAN_POINT ( 'NONE',  ( -10.29444468844919669, 9.261019486351067087, 153.1863240279699028 ) ) ;
#30288=CARTESIAN_POINT ( 'NONE',  ( 3.563940842959894884, 5.387559678655692963, 159.5815388724490163 ) ) ;
#30295=AXIS2_PLACEMENT_3D ( 'NONE', #3259, #35378, #12627 ) ;
#30300=VERTEX_POINT ( 'NONE', #9806 ) ;
#30380=CARTESIAN_POINT ( 'NONE',  ( 10.27611701369066921, 12.72178161430110066, 159.5815388724490163 ) ) ;
#30389=FACE_OUTER_BOUND ( 'NONE', #31800, .T. ) ;
#30407=DIRECTION ( 'NONE',  ( 1.000000000000000000, 0.000000000000000000, 0.000000000000000000 ) ) ;
#30412=EDGE_CURVE ( 'NONE', #3405, #15172, #34109, .T. ) ;
#30420=ORIENTED_EDGE ( 'NONE', *, *, #6437, .F. ) ;
#30431=AXIS2_PLACEMENT_3D ( 'NONE', #19973, #3805, #16788 ) ;
#30444=CARTESIAN_POINT ( 'NONE',  ( -9.036211638867925444, 5.250936033162997063, 154.4494414979812120 ) ) ;
#30448=EDGE_CURVE ( 'NONE', #2094, #4147, #37108, .T. ) ;
#30449=ORIENTED_EDGE ( 'NONE', *, *, #18806, .T. ) ;
#30450=CARTESIAN_POINT ( 'NONE',  ( 8.707710598625942211, 26.64268346825921085, 152.8454421597755015 ) ) ;
#30451=LINE ( 'NONE', #36841, #21715 ) ;
#30457=ORIENTED_EDGE ( 'NONE', *, *, #8691, .F. ) ;
#30471=ORIENTED_EDGE ( 'NONE', *, *, #6532, .T. ) ;
#30512=CARTESIAN_POINT ( 'NONE',  ( 0.000000000000000000, 17.49999999999998934, 154.5815388724490163 ) ) ;
#30520=EDGE_CURVE ( 'NONE', #18842, #4399, #37510, .T. ) ;
#30540=LINE ( 'NONE', #4173, #38063 ) ;
#30559=AXIS2_PLACEMENT_3D ( 'NONE', #4295, #4077, #20882 ) ;
#30562=ORIENTED_EDGE ( 'NONE', *, *, #375, .T. ) ;
#30565=ORIENTED_EDGE ( 'NONE', *, *, #29319, .F. ) ;
#30566=CYLINDRICAL_SURFACE ( 'NONE', #40916, 7.579174044926336506 ) ;
#30577=AXIS2_PLACEMENT_3D ( 'NONE', #6682, #19653, #7106 ) ;
#30578=DIRECTION ( 'NONE',  ( 0.000000000000000000, 0.000000000000000000, 1.000000000000000000 ) ) ;
#30580=DIRECTION ( 'NONE',  ( -0.000000000000000000, 1.000000000000000000, -0.000000000000000000 ) ) ;
#30618=VECTOR ( 'NONE', #22825, 1000.000000000000114 ) ;
#30660=CARTESIAN_POINT ( 'NONE',  ( 8.717779811041268090, 26.34707519685558097, 152.7173826728522101 ) ) ;
#30665=DIRECTION ( 'NONE',  ( -0.000000000000000000, 0.000000000000000000, 1.000000000000000000 ) ) ;
#30666=CARTESIAN_POINT ( 'NONE',  ( 7.892226332656557375, 28.77671744963969047, 153.5487751541048738 ) ) ;
#30703=CARTESIAN_POINT ( 'NONE',  ( 10.41947860041720908, 17.49999999999956302, 159.5815388724490163 ) ) ;
#30734=B_SPLINE_CURVE_WITH_KNOTS ( 'NONE', 3,
 ( #20591, #30996, #32749, #27599, #11017, #1852, #27800, #27393, #24003, #17612, #23186, #17406, #39335, #17814 ),
 .UNSPECIFIED., .F., .F.,
 ( 4, 2, 2, 2, 2, 2, 4 ),
 ( 2.503320334721363850E-07, 0.001295412938146457997, 0.001942994241202952764, 0.002590575544259447315, 0.003238156847315941649, 0.003885738150372436851, 0.005180900756485405136 ),
 .UNSPECIFIED. ) ;
#30748=LINE ( 'NONE', #1816, #908 ) ;
#30760=EDGE_LOOP ( 'NONE', ( #14140, #22926, #29988, #28959 ) ) ;
#30777=ORIENTED_EDGE ( 'NONE', *, *, #23091, .T. ) ;
#30810=DIRECTION ( 'NONE',  ( 0.4702281306424899165, 0.8825449026267555563, 0.000000000000000000 ) ) ;
#30822=CARTESIAN_POINT ( 'NONE',  ( 2.485010488553077934, 29.11408825030370906, 152.3738872082077478 ) ) ;
#30868=DIRECTION ( 'NONE',  ( 0.000000000000000000, -0.000000000000000000, -1.000000000000000000 ) ) ;
#30871=CARTESIAN_POINT ( 'NONE',  ( 10.43951711756744949, 22.06308511897971059, 152.0807009029541348 ) ) ;
#30884=LINE ( 'NONE', #1941, #2041 ) ;
#30931=DIRECTION ( 'NONE',  ( 0.8660254037844397068, -0.4999999999999979461, 0.000000000000000000 ) ) ;
#30932=AXIS2_PLACEMENT_3D ( 'NONE', #34130, #18178, #24160 ) ;
#30944=EDGE_LOOP ( 'NONE', ( #11471, #10622, #4779, #41402 ) ) ;
#30947=CYLINDRICAL_SURFACE ( 'NONE', #30932, 5.000000000000000888 ) ;
#30985=ORIENTED_EDGE ( 'NONE', *, *, #4016, .T. ) ;
#30991=DIRECTION ( 'NONE',  ( -0.000000000000000000, 0.000000000000000000, -1.000000000000000000 ) ) ;
#30995=ORIENTED_EDGE ( 'NONE', *, *, #30412, .T. ) ;
#30996=CARTESIAN_POINT ( 'NONE',  ( -13.41035298162403855, 21.52739493213463717, 153.6942049793719889 ) ) ;
#31005=ORIENTED_EDGE ( 'NONE', *, *, #25435, .F. ) ;
#31010=CARTESIAN_POINT ( 'NONE',  ( -16.28249153430137497, 8.099299129593275026, 159.5815388724490163 ) ) ;
#31020=CARTESIAN_POINT ( 'NONE',  ( 15.15544456622762759, 26.25000000000004974, 154.5815388724490163 ) ) ;
#31024=FACE_OUTER_BOUND ( 'NONE', #6085, .T. ) ;
#31042=FACE_OUTER_BOUND ( 'NONE', #30147, .T. ) ;
#31045=EDGE_LOOP ( 'NONE', ( #27383, #4245, #36042, #8937, #162, #6611 ) ) ;
#31055=CARTESIAN_POINT ( 'NONE',  ( -10.20684115509089906, 26.69374788516367403, 153.5324451153149994 ) ) ;
#31058=CARTESIAN_POINT ( 'NONE',  ( 5.079011605970033649, 4.975805295193828748, 153.3946900321003568 ) ) ;
#31070=CARTESIAN_POINT ( 'NONE',  ( -3.500000000000003997, 17.49999999999998934, 141.5815388724490163 ) ) ;
#31085=ORIENTED_EDGE ( 'NONE', *, *, #41989, .T. ) ;
#31115=DIRECTION ( 'NONE',  ( 1.000000000000000000, 0.000000000000000000, 0.000000000000000000 ) ) ;
#31141=CARTESIAN_POINT ( 'NONE',  ( 13.12951721863600874, 19.71973705675782185, 153.2716563237895002 ) ) ;
#31143=CARTESIAN_POINT ( 'NONE',  ( 0.000000000000000000, 0.000000000000000000, 164.5815388724490163 ) ) ;
#31183=ORIENTED_EDGE ( 'NONE', *, *, #32656, .F. ) ;
#31217=DIRECTION ( 'NONE',  ( -0.000000000000000000, -0.000000000000000000, -1.000000000000000000 ) ) ;
#31221=AXIS2_PLACEMENT_3D ( 'NONE', #404, #13379, #26360 ) ;
#31224=DIRECTION ( 'NONE',  ( 1.000000000000000000, 0.000000000000000000, 0.000000000000000000 ) ) ;
#31242=DIRECTION ( 'NONE',  ( 0.000000000000000000, -0.000000000000000000, -1.000000000000000000 ) ) ;
#31305=AXIS2_PLACEMENT_3D ( 'NONE', #3016, #16007, #28950 ) ;
#31330=CIRCLE ( 'NONE', #8228, 3.500000000000000444 ) ;
#31348=CARTESIAN_POINT ( 'NONE',  ( 13.38787894130366674, 19.36025875490912540, 153.3956926483656673 ) ) ;
#31354=CARTESIAN_POINT ( 'NONE',  ( 10.41947860041720908, 17.49999999999956302, 159.5815388724490163 ) ) ;
#31367=ADVANCED_FACE ( 'NONE', ( #11000 ), #10785, .T. ) ;
#31434=FACE_OUTER_BOUND ( 'NONE', #18478, .T. ) ;
#31442=AXIS2_PLACEMENT_3D ( 'NONE', #33593, #14660, #40176 ) ;
#31445=VECTOR ( 'NONE', #17912, 1000.000000000000000 ) ;
#31447=ORIENTED_EDGE ( 'NONE', *, *, #16344, .T. ) ;
#31474=CIRCLE ( 'NONE', #29435, 5.000000000000000888 ) ;
#31556=CIRCLE ( 'NONE', #4429, 5.000000000000000888 ) ;
#31591=AXIS2_PLACEMENT_3D ( 'NONE', #31354, #21155, #18385 ) ;
#31595=LINE ( 'NONE', #12237, #35481 ) ;
#31672=DIRECTION ( 'NONE',  ( 0.000000000000000000, 0.000000000000000000, 1.000000000000000000 ) ) ;
#31694=CARTESIAN_POINT ( 'NONE',  ( -8.707710598626928089, 8.357316531739312992, 152.8454421597761836 ) ) ;
#31697=EDGE_CURVE ( 'NONE', #4657, #17600, #18945, .T. ) ;
#31703=ORIENTED_EDGE ( 'NONE', *, *, #31880, .F. ) ;
#31732=CARTESIAN_POINT ( 'NONE',  ( 14.87145978460194762, 15.21432821043589634, 154.3410716200989725 ) ) ;
#31799=DIRECTION ( 'NONE',  ( -0.9994203709764782895, 0.03404294460293555424, 0.000000000000000000 ) ) ;
#31800=EDGE_LOOP ( 'NONE', ( #9069, #13189, #41136, #2523 ) ) ;
#31801=VERTEX_POINT ( 'NONE', #35833 ) ;
#31813=EDGE_CURVE ( 'NONE', #36157, #8278, #7008, .T. ) ;
#31815=CARTESIAN_POINT ( 'NONE',  ( -5.209739300209236035, 8.476466837849001124, 150.5815388724490163 ) ) ;
#31817=CARTESIAN_POINT ( 'NONE',  ( -14.96622041527907498, 15.40889182475245356, 154.3815176410583376 ) ) ;
#31829=DIRECTION ( 'NONE',  ( -1.000000000000000000, 0.000000000000000000, -0.000000000000000000 ) ) ;
#31843=VECTOR ( 'NONE', #30931, 1000.000000000000114 ) ;
#31861=CARTESIAN_POINT ( 'NONE',  ( -3.042470621311484269, 5.665403861746784564, 152.5896212286794764 ) ) ;
#31864=ORIENTED_EDGE ( 'NONE', *, *, #32867, .T. ) ;
#31868=CARTESIAN_POINT ( 'NONE',  ( 12.73238323000433425, 14.85733105118995567, 153.0776982460618569 ) ) ;
#31880=EDGE_CURVE ( 'NONE', #33258, #14205, #16493, .T. ) ;
#31912=AXIS2_PLACEMENT_3D ( 'NONE', #9786, #22744, #36345 ) ;
#31923=EDGE_CURVE ( 'NONE', #32814, #9816, #14629, .T. ) ;
#31929=CIRCLE ( 'NONE', #23824, 3.499999999999999556 ) ;
#31934=EDGE_CURVE ( 'NONE', #38421, #35160, #20733, .T. ) ;
#31941=AXIS2_PLACEMENT_3D ( 'NONE', #12735, #28676, #35493 ) ;
#32002=CARTESIAN_POINT ( 'NONE',  ( -8.745125217307586851, 8.949828348578465764, 152.5993402266566932 ) ) ;
#32027=VERTEX_POINT ( 'NONE', #40700 ) ;
#32032=ORIENTED_EDGE ( 'NONE', *, *, #27690, .T. ) ;
#32058=ORIENTED_EDGE ( 'NONE', *, *, #24561, .T. ) ;
#32072=CARTESIAN_POINT ( 'NONE',  ( -8.306764786576346538, 6.839349216201681791, 153.3946901339296289 ) ) ;
#32074=CARTESIAN_POINT ( 'NONE',  ( -7.463020515686094924, 29.21892818346099219, 153.6272566616691222 ) ) ;
#32075=DIRECTION ( 'NONE',  ( 1.000000000000000000, 0.000000000000000000, 0.000000000000000000 ) ) ;
#32078=VERTEX_POINT ( 'NONE', #24144 ) ;
#32091=DIRECTION ( 'NONE',  ( 0.000000000000000000, 0.000000000000000000, -1.000000000000000000 ) ) ;
#32152=FACE_OUTER_BOUND ( 'NONE', #6513, .T. ) ;
#32160=CARTESIAN_POINT ( 'NONE',  ( 15.36256818513868083, 16.63324207728947002, 154.5490570889038224 ) ) ;
#32173=CARTESIAN_POINT ( 'NONE',  ( -13.06543980208746447, 13.25749020988016547, 159.5815388724490163 ) ) ;
#32189=EDGE_CURVE ( 'NONE', #40356, #20414, #1444, .T. ) ;
#32225=CARTESIAN_POINT ( 'NONE',  ( 10.41947860041720375, 17.49999999999957012, 159.5815388724490163 ) ) ;
#32227=DIRECTION ( 'NONE',  ( 0.000000000000000000, 0.000000000000000000, -1.000000000000000000 ) ) ;
#32247=ORIENTED_EDGE ( 'NONE', *, *, #5964, .F. ) ;
#32262=CARTESIAN_POINT ( 'NONE',  ( -9.171506339049297907, 24.25934405745774924, 152.0807008240731477 ) ) ;
#32263=CARTESIAN_POINT ( 'NONE',  ( -1.000000000000119460, 28.78848757896615496, 159.5815388724490163 ) ) ;
#32264=DIRECTION ( 'NONE',  ( 1.000000000000000000, 0.000000000000000000, 0.000000000000000000 ) ) ;
#32269=CARTESIAN_POINT ( 'NONE',  ( 13.06543980208692091, 21.74250979011892326, 153.5324451153149710 ) ) ;
#32271=DIRECTION ( 'NONE',  ( -0.000000000000000000, -0.000000000000000000, -1.000000000000000000 ) ) ;
#32286=CARTESIAN_POINT ( 'NONE',  ( -9.292375245847971144, 29.41797201294944131, 154.3820435809088281 ) ) ;
#32289=CARTESIAN_POINT ( 'NONE',  ( -0.6348918613211859130, 28.74223512675440517, 151.9983627981021073 ) ) ;
#32291=CARTESIAN_POINT ( 'NONE',  ( -4.496074243414083682, 29.95302816219199116, 153.2247034038990705 ) ) ;
#32295=ORIENTED_EDGE ( 'NONE', *, *, #35088, .F. ) ;
#32299=AXIS2_PLACEMENT_3D ( 'NONE', #22823, #25606, #269 ) ;
#32321=FACE_OUTER_BOUND ( 'NONE', #25373, .T. ) ;
#32342=ORIENTED_EDGE ( 'NONE', *, *, #13440, .F. ) ;
#32346=EDGE_CURVE ( 'NONE', #37104, #21263, #21641, .T. ) ;
#32370=DIRECTION ( 'NONE',  ( -0.8660254037844363761, -0.5000000000000039968, 0.000000000000000000 ) ) ;
#32380=EDGE_CURVE ( 'NONE', #40356, #6293, #27799, .T. ) ;
#32419=CARTESIAN_POINT ( 'NONE',  ( -9.418615391893489175, 11.32905018158522381, 151.9983627776730373 ) ) ;
#32444=ORIENTED_EDGE ( 'NONE', *, *, #21571, .F. ) ;
#32452=EDGE_CURVE ( 'NONE', #24301, #40091, #13501, .T. ) ;
#32455=EDGE_CURVE ( 'NONE', #17339, #29598, #13368, .T. ) ;
#32466=CARTESIAN_POINT ( 'NONE',  ( -8.815590319779078143, 25.45912597582881887, 152.3738871122214960 ) ) ;
#32476=DIRECTION ( 'NONE',  ( -0.000000000000000000, -0.000000000000000000, -1.000000000000000000 ) ) ;
#32503=CARTESIAN_POINT ( 'NONE',  ( 13.91947860041721086, 17.19212016137696963, 153.6452861111154675 ) ) ;
#32508=CARTESIAN_POINT ( 'NONE',  ( 4.826850757002268288, 31.51329601944702929, 154.2021328595026830 ) ) ;
#32539=VECTOR ( 'NONE', #12079, 1000.000000000000000 ) ;
#32565=CARTESIAN_POINT ( 'NONE',  ( 9.873783753533958318, 12.15816195922839249, 151.9771749151017559 ) ) ;
#32587=DIRECTION ( 'NONE',  ( 0.000000000000000000, 0.000000000000000000, -1.000000000000000000 ) ) ;
#32621=CARTESIAN_POINT ( 'NONE',  ( -9.070267145359183658, 10.44973680043937136, 152.1397377088998724 ) ) ;
#32646=DIRECTION ( 'NONE',  ( -0.000000000000000000, -0.000000000000000000, -1.000000000000000000 ) ) ;
#32656=EDGE_CURVE ( 'NONE', #3492, #9007, #1247, .T. ) ;
#32664=TOROIDAL_SURFACE ( 'NONE', #15044, 11.07917404492494029, 5.000000000000000000 ) ;
#32669=CARTESIAN_POINT ( 'NONE',  ( -9.873783753534072005, 22.84183804077052216, 151.9771749151017843 ) ) ;
#32671=CARTESIAN_POINT ( 'NONE',  ( 2.302507646137074410E-15, -1.301401740813418195, 150.5815388724490163 ) ) ;
#32676=CARTESIAN_POINT ( 'NONE',  ( 15.41947860041720908, 17.93642350053847423, 154.5727510624242882 ) ) ;
#32684=ORIENTED_EDGE ( 'NONE', *, *, #5785, .F. ) ;
#32700=LINE ( 'NONE', #3362, #12406 ) ;
#32714=CARTESIAN_POINT ( 'NONE',  ( 5.675078561235607388, 31.50641906547725668, 154.3820435211242454 ) ) ;
#32730=DIRECTION ( 'NONE',  ( 0.000000000000000000, 0.000000000000000000, -1.000000000000000000 ) ) ;
#32736=CARTESIAN_POINT ( 'NONE',  ( 0.000000000000000000, 17.49999999999998934, 155.5815388724490163 ) ) ;
#32749=CARTESIAN_POINT ( 'NONE',  ( -13.72762536464784411, 21.27191211082971734, 153.8384576237823183 ) ) ;
#32814=VERTEX_POINT ( 'NONE', #18866 ) ;
#32816=DIRECTION ( 'NONE',  ( 1.000000000000000000, 0.000000000000000000, 0.000000000000000000 ) ) ;
#32840=ADVANCED_FACE ( 'NONE', ( #25254 ), #28227, .T. ) ;
#32843=CARTESIAN_POINT ( 'NONE',  ( -13.91947860041774376, 17.49999999999951683, 153.6452861111158086 ) ) ;
#32845=ORIENTED_EDGE ( 'NONE', *, *, #39714, .F. ) ;
#32858=AXIS2_PLACEMENT_3D ( 'NONE', #40850, #11703, #37663 ) ;
#32867=EDGE_CURVE ( 'NONE', #3492, #16759, #2284, .T. ) ;
#32870=DIRECTION ( 'NONE',  ( 1.000000000000000000, 0.000000000000000000, 0.000000000000000000 ) ) ;
#32885=CARTESIAN_POINT ( 'NONE',  ( 14.87346161161427283, 19.78183385133235106, 154.3419292312980815 ) ) ;
#32903=CARTESIAN_POINT ( 'NONE',  ( -9.888348281642997506, 28.29975245075289791, 154.0918075026113740 ) ) ;
#32906=EDGE_CURVE ( 'NONE', #16970, #21296, #38220, .T. ) ;
#32915=ORIENTED_EDGE ( 'NONE', *, *, #36770, .F. ) ;
#32928=EDGE_CURVE ( 'NONE', #5194, #6594, #5089, .T. ) ;
#32955=ADVANCED_FACE ( 'NONE', ( #2492 ), #27811, .F. ) ;
#32972=ORIENTED_EDGE ( 'NONE', *, *, #36770, .T. ) ;
#32984=LINE ( 'NONE', #27458, #40912 ) ;
#32993=EDGE_CURVE ( 'NONE', #11324, #28722, #35032, .T. ) ;
#33001=EDGE_LOOP ( 'NONE', ( #17433, #12280, #37255, #36263 ) ) ;
#33021=DIRECTION ( 'NONE',  ( 1.000000000000000000, 0.000000000000000000, 0.000000000000000000 ) ) ;
#33045=CARTESIAN_POINT ( 'NONE',  ( 9.718734271692364146, 11.88888615205621946, 159.5815388724490163 ) ) ;
#33058=ORIENTED_EDGE ( 'NONE', *, *, #40159, .T. ) ;
#33094=CARTESIAN_POINT ( 'NONE',  ( 10.36407707418830171, 9.510225563413008842, 153.1288290536735133 ) ) ;
#33127=ORIENTED_EDGE ( 'NONE', *, *, #23433, .T. ) ;
#33128=EDGE_CURVE ( 'NONE', #5552, #20998, #7821, .T. ) ;
#33151=ORIENTED_EDGE ( 'NONE', *, *, #2193, .T. ) ;
#33162=ORIENTED_EDGE ( 'NONE', *, *, #36280, .T. ) ;
#33182=ORIENTED_EDGE ( 'NONE', *, *, #712, .F. ) ;
#33204=CARTESIAN_POINT ( 'NONE',  ( -12.27165144158644061, 20.46975685308312976, 159.5815388724490163 ) ) ;
#33205=CARTESIAN_POINT ( 'NONE',  ( -3.603329285779699021, 3.723597269576835345, 153.8406024308892768 ) ) ;
#33210=ORIENTED_EDGE ( 'NONE', *, *, #27567, .F. ) ;
#33219=CARTESIAN_POINT ( 'NONE',  ( 10.29444468844837601, 25.73898051364774631, 153.1863240279694480 ) ) ;
#33231=DIRECTION ( 'NONE',  ( -1.000000000000000000, 0.000000000000000000, 0.000000000000000000 ) ) ;
#33246=VECTOR ( 'NONE', #489, 1000.000000000000000 ) ;
#33253=DIRECTION ( 'NONE',  ( -1.000000000000000000, 0.000000000000000000, 0.000000000000000000 ) ) ;
#33254=DIRECTION ( 'NONE',  ( -0.000000000000000000, -0.000000000000000000, -1.000000000000000000 ) ) ;
#33258=VERTEX_POINT ( 'NONE', #36281 ) ;
#33262=DIRECTION ( 'NONE',  ( 0.000000000000000000, 0.000000000000000000, 1.000000000000000000 ) ) ;
#33286=FACE_OUTER_BOUND ( 'NONE', #6710, .T. ) ;
#33316=VECTOR ( 'NONE', #9810, 1000.000000000000000 ) ;
#33329=ORIENTED_EDGE ( 'NONE', *, *, #40939, .F. ) ;
#33368=DIRECTION ( 'NONE',  ( -1.000000000000000000, 0.000000000000000000, 0.000000000000000000 ) ) ;
#33377=DIRECTION ( 'NONE',  ( -1.000000000000000000, 0.000000000000000000, 0.000000000000000000 ) ) ;
#33415=CARTESIAN_POINT ( 'NONE',  ( 10.05350722043614375, 12.42871502819271434, 151.9983628076606408 ) ) ;
#33424=CARTESIAN_POINT ( 'NONE',  ( -8.435140907415922484, 4.631751190418449404, 154.5487361196980771 ) ) ;
#33447=CARTESIAN_POINT ( 'NONE',  ( -10.77809958360008658, 24.30802190437292509, 152.9195735126124873 ) ) ;
#33448=CARTESIAN_POINT ( 'NONE',  ( -10.20684115509165224, 8.306252114835194433, 153.5324451153154826 ) ) ;
#33449=AXIS2_PLACEMENT_3D ( 'NONE', #41737, #22367, #15794 ) ;
#33483=AXIS2_PLACEMENT_3D ( 'NONE', #24027, #24439, #37203 ) ;
#33510=CARTESIAN_POINT ( 'NONE',  ( -10.53587323178440194, 22.42818870813906429, 154.5815388724490163 ) ) ;
#33522=CARTESIAN_POINT ( 'NONE',  ( -16.28249153430137852, 26.90070087040669478, 150.5815388724490163 ) ) ;
#33552=CIRCLE ( 'NONE', #26776, 5.000000000000000000 ) ;
#33555=CARTESIAN_POINT ( 'NONE',  ( -8.486615222244203949, 27.76195273331519431, 153.2720929549179800 ) ) ;
#33559=ORIENTED_EDGE ( 'NONE', *, *, #5250, .F. ) ;
#33589=DIRECTION ( 'NONE',  ( -1.000000000000000000, 0.000000000000000000, 0.000000000000000000 ) ) ;
#33591=ORIENTED_EDGE ( 'NONE', *, *, #7991, .T. ) ;
#33593=CARTESIAN_POINT ( 'NONE',  ( 0.000000000000000000, 17.49999999999998934, 150.5815388724490163 ) ) ;
#33598=EDGE_CURVE ( 'NONE', #18842, #6127, #15986, .T. ) ;
#33604=ORIENTED_EDGE ( 'NONE', *, *, #14525, .T. ) ;
#33648=CARTESIAN_POINT ( 'NONE',  ( -8.092379817709877798, 4.367781802507559874, 154.5725613230242175 ) ) ;
#33677=CIRCLE ( 'NONE', #26869, 6.079174044926337395 ) ;
#33688=EDGE_CURVE ( 'NONE', #17600, #19866, #15636, .T. ) ;
#33695=CARTESIAN_POINT ( 'NONE',  ( -12.28618350919750668, 12.68681765321529831, 153.1965160676645041 ) ) ;
#33725=DIRECTION ( 'NONE',  ( -1.000000000000000000, 0.000000000000000000, 0.000000000000000000 ) ) ;
#33779=LINE ( 'NONE', #4635, #40718 ) ;
#33798=FACE_OUTER_BOUND ( 'NONE', #9409, .T. ) ;
#33833=DIRECTION ( 'NONE',  ( -0.000000000000000000, 0.000000000000000000, 1.000000000000000000 ) ) ;
#33847=CARTESIAN_POINT ( 'NONE',  ( -5.039920647268967713, 3.474869008664458914, 154.2527047512478191 ) ) ;
#33852=CARTESIAN_POINT ( 'NONE',  ( 9.070267145358528182, 24.55026319955927505, 152.1397377088993608 ) ) ;
#33855=VERTEX_POINT ( 'NONE', #7526 ) ;
#33857=CARTESIAN_POINT ( 'NONE',  ( 8.306764786575204340, 28.16065078379654452, 153.3946901339287194 ) ) ;
#33916=DIRECTION ( 'NONE',  ( -1.000000000000000000, 0.000000000000000000, 0.000000000000000000 ) ) ;
#33940=CARTESIAN_POINT ( 'NONE',  ( -12.27165144158654719, 14.53024314691597141, 159.5815388724490163 ) ) ;
#33954=AXIS2_PLACEMENT_3D ( 'NONE', #29502, #26539, #23564 ) ;
#33962=ORIENTED_EDGE ( 'NONE', *, *, #10599, .F. ) ;
#33968=EDGE_CURVE ( 'NONE', #8699, #6127, #41112, .T. ) ;
#33989=PRODUCT_DEFINITION_SHAPE ( 'NONE', 'NONE',  #8844 ) ;
#34009=EDGE_CURVE ( 'NONE', #29125, #29783, #39073, .T. ) ;
#34015=DIRECTION ( 'NONE',  ( -1.000000000000000000, 0.000000000000000000, 0.000000000000000000 ) ) ;
#34019=ADVANCED_FACE ( 'NONE', ( #34510 ), #5368, .F. ) ;
#34022=ORIENTED_EDGE ( 'NONE', *, *, #10953, .T. ) ;
#34109=LINE ( 'NONE', #21136, #11442 ) ;
#34117=ORIENTED_EDGE ( 'NONE', *, *, #41989, .F. ) ;
#34130=CARTESIAN_POINT ( 'NONE',  ( -10.41947860041774199, 17.49999999999951683, 150.5815388724490163 ) ) ;
#34163=SPHERICAL_SURFACE ( 'NONE', #9762, 5.000000000000000000 ) ;
#34172=EDGE_LOOP ( 'NONE', ( #35251, #19612, #35531, #15143 ) ) ;
#34175=( NAMED_UNIT ( * ) PLANE_ANGLE_UNIT ( ) SI_UNIT ( $, .RADIAN. ) );
#34195=DIRECTION ( 'NONE',  ( -1.000000000000000000, 0.000000000000000000, 0.000000000000000000 ) ) ;
#34211=FACE_OUTER_BOUND ( 'NONE', #41342, .T. ) ;
#34228=VECTOR ( 'NONE', #40853, 1000.000000000000000 ) ;
#34230=EDGE_CURVE ( 'NONE', #38078, #18650, #33677, .T. ) ;
#34292=CIRCLE ( 'NONE', #5757, 5.000000000000000888 ) ;
#34320=CARTESIAN_POINT ( 'NONE',  ( 2.302507646137074410E-15, -1.301401740813418195, 159.5815388724490163 ) ) ;
#34333=ORIENTED_EDGE ( 'NONE', *, *, #40701, .F. ) ;
#34339=AXIS2_PLACEMENT_3D ( 'NONE', #1464, #10617, #1050 ) ;
#34343=CARTESIAN_POINT ( 'NONE',  ( -16.28249153430137497, 8.099299129593275026, 159.5815388724490163 ) ) ;
#34386=FACE_OUTER_BOUND ( 'NONE', #27391, .T. ) ;
#34391=CARTESIAN_POINT ( 'NONE',  ( -14.87346161161482172, 15.21816614866675899, 154.3419292312983941 ) ) ;
#34402=CARTESIAN_POINT ( 'NONE',  ( 0.000000000000000000, 17.49999999999998934, 155.5815388724490163 ) ) ;
#34417=ORIENTED_EDGE ( 'NONE', *, *, #32346, .F. ) ;
#34418=EDGE_CURVE ( 'NONE', #37892, #28523, #364, .T. ) ;
#34426=CARTESIAN_POINT ( 'NONE',  ( -4.330127018922124371, 14.99999999999985789, 159.5815388724490163 ) ) ;
#34453=CARTESIAN_POINT ( 'NONE',  ( 5.970050184155318185, 5.056703826249529854, 153.5717503611256802 ) ) ;
#34455=EDGE_CURVE ( 'NONE', #36157, #21296, #21024, .T. ) ;
#34478=ORIENTED_EDGE ( 'NONE', *, *, #37656, .F. ) ;
#34507=FACE_OUTER_BOUND ( 'NONE', #19578, .T. ) ;
#34510=FACE_OUTER_BOUND ( 'NONE', #41606, .T. ) ;
#34521=ORIENTED_EDGE ( 'NONE', *, *, #27932, .T. ) ;
#34526=DIRECTION ( 'NONE',  ( -1.000000000000000000, 0.000000000000000000, 0.000000000000000000 ) ) ;
#34574=CARTESIAN_POINT ( 'NONE',  ( 10.20684115509066103, 26.69374788516360297, 159.5815388724490163 ) ) ;
#34589=ORIENTED_EDGE ( 'NONE', *, *, #37656, .T. ) ;
#34594=CARTESIAN_POINT ( 'NONE',  ( -15.41947860041774376, 17.49999999999951683, 159.5815388724490163 ) ) ;
#34596=DIRECTION ( 'NONE',  ( -0.000000000000000000, -0.000000000000000000, 1.000000000000000000 ) ) ;
#34606=CIRCLE ( 'NONE', #3373, 7.579174044926336506 ) ;
#34619=CARTESIAN_POINT ( 'NONE',  ( 1.196959198423996895E-13, 5.911571776152701574, 154.5815388724490163 ) ) ;
#34622=AXIS2_PLACEMENT_3D ( 'NONE', #17276, #40235, #1114 ) ;
#34636=DIRECTION ( 'NONE',  ( 0.8485019580238700732, -0.5291922403339439640, 0.000000000000000000 ) ) ;
#34660=CARTESIAN_POINT ( 'NONE',  ( 8.707710598626619003, 8.357316531739469312, 152.8454421597759847 ) ) ;
#34675=CARTESIAN_POINT ( 'NONE',  ( -5.209739300208505064, 26.52353316214900047, 159.5815388724490163 ) ) ;
#34756=DIRECTION ( 'NONE',  ( -1.000000000000000000, 0.000000000000000000, 0.000000000000000000 ) ) ;
#34771=EDGE_CURVE ( 'NONE', #4262, #40121, #5272, .T. ) ;
#34813=CIRCLE ( 'NONE', #17153, 5.000000000000000000 ) ;
#34817=AXIS2_PLACEMENT_3D ( 'NONE', #15034, #28208, #21409 ) ;
#34820=DIRECTION ( 'NONE',  ( 0.000000000000000000, 0.000000000000000000, 1.000000000000000000 ) ) ;
#34850=EDGE_LOOP ( 'NONE', ( #7442, #29992, #31183, #31864 ) ) ;
#34853=CARTESIAN_POINT ( 'NONE',  ( -10.41947860041774199, 17.49999999999951683, 159.5815388724490163 ) ) ;
#34881=CARTESIAN_POINT ( 'NONE',  ( 4.330127018922108384, 20.00000000000014211, 159.5815388724490163 ) ) ;
#34929=DIRECTION ( 'NONE',  ( -0.000000000000000000, -0.000000000000000000, 1.000000000000000000 ) ) ;
#34945=CARTESIAN_POINT ( 'NONE',  ( 2.858598646995994308, 4.063742324715648557, 153.5324451153153973 ) ) ;
#34961=ADVANCED_FACE ( 'NONE', ( #9518 ), #13125, .T. ) ;
#34962=CARTESIAN_POINT ( 'NONE',  ( 10.20684115509065926, 26.69374788516359942, 153.5324451153148573 ) ) ;
#34969=ADVANCED_FACE ( 'NONE', ( #42063 ), #7166, .F. ) ;
#34988=DIRECTION ( 'NONE',  ( -0.8660254037844363761, -0.5000000000000039968, 0.000000000000000000 ) ) ;
#35007=AXIS2_PLACEMENT_3D ( 'NONE', #14542, #21542, #11337 ) ;
#35031=VECTOR ( 'NONE', #14522, 1000.000000000000000 ) ;
#35032=LINE ( 'NONE', #5262, #1698 ) ;
#35059=ORIENTED_EDGE ( 'NONE', *, *, #18154, .F. ) ;
#35062=DIRECTION ( 'NONE',  ( -0.5291922403339439640, -0.8485019580238700732, 0.000000000000000000 ) ) ;
#35088=EDGE_CURVE ( 'NONE', #2798, #5194, #20064, .T. ) ;
#35117=FACE_OUTER_BOUND ( 'NONE', #9480, .T. ) ;
#35160=VERTEX_POINT ( 'NONE', #29400 ) ;
#35196=CIRCLE ( 'NONE', #37901, 6.079174044925958142 ) ;
#35223=CARTESIAN_POINT ( 'NONE',  ( -13.40983285079620302, 13.47228067356521031, 153.6939610446748929 ) ) ;
#35238=CARTESIAN_POINT ( 'NONE',  ( 5.209739300208924284, 8.476466837849175207, 159.5815388724490163 ) ) ;
#35251=ORIENTED_EDGE ( 'NONE', *, *, #31934, .T. ) ;
#35265=EDGE_CURVE ( 'NONE', #4470, #28523, #40472, .T. ) ;
#35266=CARTESIAN_POINT ( 'NONE',  ( -0.3107243566309055849, 28.72186657361018902, 151.9771749059762556 ) ) ;
#35268=CARTESIAN_POINT ( 'NONE',  ( -6.689291174883642555, 29.71030723676863516, 153.6451024763353814 ) ) ;
#35269=CARTESIAN_POINT ( 'NONE',  ( 3.302902078253401541, 5.526643559813305018, 152.7173827288302448 ) ) ;
#35275=CARTESIAN_POINT ( 'NONE',  ( 12.27165144158615284, 14.53024314691610641, 152.8454421597757289 ) ) ;
#35286=EDGE_CURVE ( 'NONE', #9160, #19866, #6394, .T. ) ;
#35300=DIRECTION ( 'NONE',  ( -1.000000000000000000, 0.000000000000000000, 0.000000000000000000 ) ) ;
#35324=ORIENTED_EDGE ( 'NONE', *, *, #14001, .F. ) ;
#35346=VECTOR ( 'NONE', #37268, 1000.000000000000000 ) ;
#35350=CARTESIAN_POINT ( 'NONE',  ( 14.96450702994059334, 15.40506357400320070, 154.3807879069779574 ) ) ;
#35375=EDGE_LOOP ( 'NONE', ( #20478, #12731, #35059, #19785 ) ) ;
#35378=DIRECTION ( 'NONE',  ( 0.000000000000000000, -1.000000000000000000, 0.000000000000000000 ) ) ;
#35382=CARTESIAN_POINT ( 'NONE',  ( 9.276117013689805901, 24.01026919326780629, 159.5815388724490163 ) ) ;
#35406=CARTESIAN_POINT ( 'NONE',  ( -9.883105000805873175, 12.17284242645979297, 151.9779334031987901 ) ) ;
#35413=AXIS2_PLACEMENT_3D ( 'NONE', #14993, #20757, #14368 ) ;
#35429=B_SPLINE_CURVE_WITH_KNOTS ( 'NONE', 3,
 ( #17525, #1359, #30280, #1153, #36453, #30065, #4754, #17319, #39635, #26888, #27096, #37099, #33695, #14121, #40064, #29856 ),
 .UNSPECIFIED., .F., .F.,
 ( 4, 2, 2, 2, 2, 2, 2, 4 ),
 ( 2.129600427321431082E-07, 0.001523388048537073535, 0.002284975592784235180, 0.003046563137031397042, 0.003808150681278559338, 0.004569738225525720766, 0.005331325769772882195, 0.006092913314020044491 ),
 .UNSPECIFIED. ) ;
#35431=ORIENTED_EDGE ( 'NONE', *, *, #2744, .F. ) ;
#35432=CARTESIAN_POINT ( 'NONE',  ( 10.03587323178420476, 23.29421411192385349, 154.5815388724490163 ) ) ;
#35452=CARTESIAN_POINT ( 'NONE',  ( -9.535873231784242066, 10.83976048429175520, 154.5815388724490163 ) ) ;
#35459=CARTESIAN_POINT ( 'NONE',  ( -13.71305093447513102, 18.69374200302473454, 153.5492497259778304 ) ) ;
#35476=CARTESIAN_POINT ( 'NONE',  ( -5.453575347710231114, 31.52202144991315791, 154.3405383141641209 ) ) ;
#35481=VECTOR ( 'NONE', #30258, 1000.000000000000000 ) ;
#35482=CARTESIAN_POINT ( 'NONE',  ( -4.935610658065916034, 4.984124879058972724, 153.3570253102932384 ) ) ;
#35493=DIRECTION ( 'NONE',  ( 1.000000000000000000, 0.000000000000000000, 0.000000000000000000 ) ) ;
#35504=LINE ( 'NONE', #41680, #30223 ) ;
#35531=ORIENTED_EDGE ( 'NONE', *, *, #1604, .F. ) ;
#35547=EDGE_CURVE ( 'NONE', #26911, #11650, #21929, .T. ) ;
#35587=DIRECTION ( 'NONE',  ( -1.000000000000000000, 0.000000000000000000, 0.000000000000000000 ) ) ;
#35601=AXIS2_PLACEMENT_3D ( 'NONE', #17485, #30868, #14905 ) ;
#35643=ORIENTED_EDGE ( 'NONE', *, *, #25136, .T. ) ;
#35660=FACE_OUTER_BOUND ( 'NONE', #16710, .T. ) ;
#35666=CARTESIAN_POINT ( 'NONE',  ( -8.727825599366182630, 26.05215460137525341, 152.5896210917537985 ) ) ;
#35673=CARTESIAN_POINT ( 'NONE',  ( 11.14833699762147035, 11.36451542402420145, 152.9052493666960117 ) ) ;
#35681=VERTEX_POINT ( 'NONE', #5347 ) ;
#35700=ORIENTED_EDGE ( 'NONE', *, *, #14471, .F. ) ;
#35703=CARTESIAN_POINT ( 'NONE',  ( 13.59845369259831926, 16.02800949298296018, 153.4954411043902667 ) ) ;
#35736=EDGE_LOOP ( 'NONE', ( #14575, #23890, #40233, #6811, #38146, #26819, #15458, #28623 ) ) ;
#35739=ADVANCED_FACE ( 'NONE', ( #35117 ), #2578, .T. ) ;
#35757=STYLED_ITEM('',(#42159),#36847);
#35768=CARTESIAN_POINT ( 'NONE',  ( 9.171506339049368961, 10.74065594254105527, 152.0807008240732614 ) ) ;
#35782=DIRECTION ( 'NONE',  ( -0.000000000000000000, -0.000000000000000000, 1.000000000000000000 ) ) ;
#35787=CARTESIAN_POINT ( 'NONE',  ( 10.22308315533724077, 26.21692115641960186, 153.3425882844784383 ) ) ;
#35820=CARTESIAN_POINT ( 'NONE',  ( -10.43951711756793443, 12.93691488101921827, 152.0807009029544474 ) ) ;
#35833=CARTESIAN_POINT ( 'NONE',  ( 13.06543980208709499, 13.25749020988031823, 153.5324451153150562 ) ) ;
#35841=ORIENTED_EDGE ( 'NONE', *, *, #23105, .F. ) ;
#35846=CARTESIAN_POINT ( 'NONE',  ( 10.20684115509134315, 8.306252114835306344, 159.5815388724490163 ) ) ;
#35862=LINE ( 'NONE', #28644, #40315 ) ;
#35868=CARTESIAN_POINT ( 'NONE',  ( 11.59276877416546725, 11.97566355480205580, 152.9774434186093686 ) ) ;
#35881=CARTESIAN_POINT ( 'NONE',  ( -10.03587323178424562, 11.70578588807619091, 154.5815388724490163 ) ) ;
#35898=DIRECTION ( 'NONE',  ( 1.000000000000000000, 0.000000000000000000, 0.000000000000000000 ) ) ;
#35908=CARTESIAN_POINT ( 'NONE',  ( 4.408685582964912086, 31.46343700237504137, 154.0918074332469700 ) ) ;
#35918=FACE_OUTER_BOUND ( 'NONE', #24818, .T. ) ;
#35931=CARTESIAN_POINT ( 'NONE',  ( -1.261328688602880943, 30.34926828898636231, 153.0204462508472147 ) ) ;
#35963=CIRCLE ( 'NONE', #5127, 3.500000000000003997 ) ;
#35970=CARTESIAN_POINT ( 'NONE',  ( -5.209739300209236035, 8.476466837849001124, 159.5815388724490163 ) ) ;
#35978=ORIENTED_EDGE ( 'NONE', *, *, #29829, .T. ) ;
#35986=EDGE_CURVE ( 'NONE', #9160, #21296, #30734, .T. ) ;
#36015=EDGE_CURVE ( 'NONE', #36248, #26696, #14630, .T. ) ;
#36025=B_SPLINE_CURVE_WITH_KNOTS ( 'NONE', 3,
 ( #25459, #2689, #22047, #5883, #18854, #31817, #34391, #8860, #15041, #38422, #2272, #28836, #35223, #18652 ),
 .UNSPECIFIED., .F., .F.,
 ( 4, 2, 2, 2, 2, 2, 4 ),
 ( 0.005180900756485405136, 0.006473513313900876830, 0.007119819592608617881, 0.007766125871316353728, 0.008412432150024089575, 0.009058738428731826289, 0.01035135098614732227 ),
 .UNSPECIFIED. ) ;
#36042=ORIENTED_EDGE ( 'NONE', *, *, #26881, .T. ) ;
#36093=CARTESIAN_POINT ( 'NONE',  ( -9.030446397028269345, 29.75585273266821673, 154.4507089031951921 ) ) ;
#36121=DIRECTION ( 'NONE',  ( -1.000000000000000000, 0.000000000000000000, 0.000000000000000000 ) ) ;
#36146=ORIENTED_EDGE ( 'NONE', *, *, #36254, .T. ) ;
#36157=VERTEX_POINT ( 'NONE', #21209 ) ;
#36181=CARTESIAN_POINT ( 'NONE',  ( -6.098656404398085762, 3.551477605848323282, 154.4507088739399023 ) ) ;
#36204=CARTESIAN_POINT ( 'NONE',  ( -10.23713785027242196, 26.21549807514553265, 153.3506917991487342 ) ) ;
#36224=EDGE_CURVE ( 'NONE', #21296, #10736, #36025, .T. ) ;
#36232=CYLINDRICAL_SURFACE ( 'NONE', #9759, 3.500000000000000444 ) ;
#36248=VERTEX_POINT ( 'NONE', #5252 ) ;
#36254=EDGE_CURVE ( 'NONE', #27377, #4262, #21620, .T. ) ;
#36262=LINE ( 'NONE', #41833, #19076 ) ;
#36263=ORIENTED_EDGE ( 'NONE', *, *, #32993, .T. ) ;
#36268=CARTESIAN_POINT ( 'NONE',  ( 3.563940842959894884, 5.387559678655694739, 152.8454421597760700 ) ) ;
#36280=EDGE_CURVE ( 'NONE', #7452, #11324, #15373, .T. ) ;
#36281=CARTESIAN_POINT ( 'NONE',  ( 12.27165144158600363, 20.46975685308311554, 159.5815388724490163 ) ) ;
#36289=CARTESIAN_POINT ( 'NONE',  ( 15.19729569207780173, 18.98967089442418299, 154.4794923609102568 ) ) ;
#36296=DIRECTION ( 'NONE',  ( -1.000000000000000000, 0.000000000000000000, 0.000000000000000000 ) ) ;
#36311=ORIENTED_EDGE ( 'NONE', *, *, #16166, .F. ) ;
#36312=ORIENTED_EDGE ( 'NONE', *, *, #8177, .T. ) ;
#36313=VECTOR ( 'NONE', #9736, 1000.000000000000000 ) ;
#36327=CIRCLE ( 'NONE', #18662, 6.079174044924941178 ) ;
#36345=DIRECTION ( 'NONE',  ( -1.000000000000000000, 0.000000000000000000, 0.000000000000000000 ) ) ;
#36370=PRODUCT_DEFINITION_FORMATION_WITH_SPECIFIED_SOURCE ( 'ANY', '', #27193, .NOT_KNOWN. ) ;
#36376=ORIENTED_EDGE ( 'NONE', *, *, #26881, .F. ) ;
#36381=ORIENTED_EDGE ( 'NONE', *, *, #32455, .T. ) ;
#36401=DIRECTION ( 'NONE',  ( -0.000000000000000000, -0.000000000000000000, -1.000000000000000000 ) ) ;
#36410=CARTESIAN_POINT ( 'NONE',  ( 12.27165144158600185, 20.46975685308311554, 152.8454421597756436 ) ) ;
#36413=ORIENTED_EDGE ( 'NONE', *, *, #2957, .T. ) ;
#36429=DIRECTION ( 'NONE',  ( 0.000000000000000000, 0.000000000000000000, -1.000000000000000000 ) ) ;
#36453=CARTESIAN_POINT ( 'NONE',  ( -10.58060021646055837, 10.22253632205953622, 152.9774433574592081 ) ) ;
#36494=LINE ( 'NONE', #40527, #29256 ) ;
#36513=ORIENTED_EDGE ( 'NONE', *, *, #19993, .T. ) ;
#36534=CARTESIAN_POINT ( 'NONE',  ( -1.000000000000119460, 28.78848757896615496, 159.5815388724490163 ) ) ;
#36564=DIRECTION ( 'NONE',  ( 0.000000000000000000, 0.000000000000000000, -1.000000000000000000 ) ) ;
#36575=ORIENTED_EDGE ( 'NONE', *, *, #26480, .F. ) ;
#36606=DIRECTION ( 'NONE',  ( -0.000000000000000000, -0.000000000000000000, -1.000000000000000000 ) ) ;
#36609=ADVANCED_FACE ( 'NONE', ( #11668 ), #37835, .T. ) ;
#36625=CARTESIAN_POINT ( 'NONE',  ( 8.901842255143360916, 25.14948583533392679, 152.2937014009048937 ) ) ;
#36626=CARTESIAN_POINT ( 'NONE',  ( 4.082076315226191632, 29.84938299238654480, 153.0794453411707821 ) ) ;
#36634=CARTESIAN_POINT ( 'NONE',  ( 10.49712838360395217, 25.01697694695339536, 153.0204462789262152 ) ) ;
#36640=CARTESIAN_POINT ( 'NONE',  ( -10.36407707418804947, 25.48977443658596798, 153.1288290536733427 ) ) ;
#36650=DIRECTION ( 'NONE',  ( 1.000000000000000000, 0.000000000000000000, 0.000000000000000000 ) ) ;
#36678=CARTESIAN_POINT ( 'NONE',  ( -12.27165144158654542, 14.53024314691596963, 152.8454421597759563 ) ) ;
#36711=DIRECTION ( 'NONE',  ( 0.000000000000000000, 0.000000000000000000, 1.000000000000000000 ) ) ;
#36725=AXIS2_PLACEMENT_3D ( 'NONE', #33510, #17353, #16515 ) ;
#36765=DIRECTION ( 'NONE',  ( -1.000000000000000000, 0.000000000000000000, 0.000000000000000000 ) ) ;
#36770=EDGE_CURVE ( 'NONE', #18422, #8117, #18480, .T. ) ;
#36776=PLANE ( 'NONE',  #20361 ) ;
#36778=ORIENTED_EDGE ( 'NONE', *, *, #1693, .T. ) ;
#36781=LINE ( 'NONE', #36999, #4269 ) ;
#36792=AXIS2_PLACEMENT_3D ( 'NONE', #31010, #2493, #6530 ) ;
#36804=DIRECTION ( 'NONE',  ( 0.000000000000000000, -1.000000000000000000, 0.000000000000000000 ) ) ;
#36805=ADVANCED_FACE ( 'NONE', ( #16354 ), #9765, .T. ) ;
#36841=CARTESIAN_POINT ( 'NONE',  ( 1.196959198423996895E-13, 5.911571776152701574, 154.5815388724490163 ) ) ;
#36847=MANIFOLD_SOLID_BREP ( 'Cut-Revolve1', #20615 ) ;
#36858=CARTESIAN_POINT ( 'NONE',  ( -12.66061713743933481, 21.99498889263267642, 153.3425884699746575 ) ) ;
#36898=CARTESIAN_POINT ( 'NONE',  ( -0.5068703235618262637, 4.761880988878413490, 152.9195735263554070 ) ) ;
#36907=CARTESIAN_POINT ( 'NONE',  ( 1.196959198423996895E-13, 12.49999999999998401, 154.5815388724490163 ) ) ;
#36932=ADVANCED_FACE ( 'NONE', ( #1439 ), #17188, .F. ) ;
#36958=AXIS2_PLACEMENT_3D ( 'NONE', #21698, #7910, #40230 ) ;
#36974=DIRECTION ( 'NONE',  ( -0.000000000000000000, -0.000000000000000000, -1.000000000000000000 ) ) ;
#36999=CARTESIAN_POINT ( 'NONE',  ( -9.718734271692440529, 11.88888615205571320, 159.5815388724490163 ) ) ;
#37002=CARTESIAN_POINT ( 'NONE',  ( 16.28249153430137852, 26.90070087040669122, 150.5815388724490163 ) ) ;
#37004=PLANE ( 'NONE',  #14425 ) ;
#37018=FACE_OUTER_BOUND ( 'NONE', #24458, .T. ) ;
#37025=ORIENTED_EDGE ( 'NONE', *, *, #23944, .F. ) ;
#37036=PLANE ( 'NONE',  #8334 ) ;
#37059=CARTESIAN_POINT ( 'NONE',  ( 3.563940842959631539, 29.61244032134256088, 152.8454421597755299 ) ) ;
#37060=VECTOR ( 'NONE', #11440, 1000.000000000000000 ) ;
#37099=CARTESIAN_POINT ( 'NONE',  ( -12.10138637141935725, 12.51933337008317970, 153.1288291267221098 ) ) ;
#37103=EDGE_CURVE ( 'NONE', #16970, #5451, #8586, .T. ) ;
#37104=VERTEX_POINT ( 'NONE', #25454 ) ;
#37108=LINE ( 'NONE', #5183, #6012 ) ;
#37166=ORIENTED_EDGE ( 'NONE', *, *, #6896, .T. ) ;
#37172=ORIENTED_EDGE ( 'NONE', *, *, #13485, .F. ) ;
#37189=FACE_OUTER_BOUND ( 'NONE', #7192, .T. ) ;
#37200=DIRECTION ( 'NONE',  ( 0.8825449026267555563, -0.4702281306424899165, 0.000000000000000000 ) ) ;
#37203=DIRECTION ( 'NONE',  ( -1.000000000000000000, 0.000000000000000000, -0.000000000000000000 ) ) ;
#37211=EDGE_LOOP ( 'NONE', ( #14002, #30777, #6911, #36381 ) ) ;
#37235=CARTESIAN_POINT ( 'NONE',  ( 8.707710598625942211, 26.64268346825921085, 159.5815388724490163 ) ) ;
#37238=CARTESIAN_POINT ( 'NONE',  ( -5.209739300209236035, 8.476466837849001124, 159.5815388724490163 ) ) ;
#37255=ORIENTED_EDGE ( 'NONE', *, *, #17404, .T. ) ;
#37268=DIRECTION ( 'NONE',  ( 0.000000000000000000, 0.000000000000000000, 1.000000000000000000 ) ) ;
#37362=ADVANCED_FACE ( 'NONE', ( #22669 ), #29041, .F. ) ;
#37391=FACE_OUTER_BOUND ( 'NONE', #14137, .T. ) ;
#37393=CARTESIAN_POINT ( 'NONE',  ( 3.563940842959628874, 29.61244032134256088, 159.5815388724490163 ) ) ;
#37406=DIRECTION ( 'NONE',  ( 0.000000000000000000, 0.000000000000000000, 1.000000000000000000 ) ) ;
#37420=EDGE_LOOP ( 'NONE', ( #1230, #32444, #35643, #813, #24720, #28084, #5354 ) ) ;
#37431=EDGE_LOOP ( 'NONE', ( #32247, #11811, #31447, #4252 ) ) ;
#37459=CYLINDRICAL_SURFACE ( 'NONE', #32858, 5.000000000000000000 ) ;
#37499=DIRECTION ( 'NONE',  ( -0.000000000000000000, 0.000000000000000000, 1.000000000000000000 ) ) ;
#37509=CYLINDRICAL_SURFACE ( 'NONE', #40740, 7.579174044925481191 ) ;
#37510=LINE ( 'NONE', #30288, #39359 ) ;
#37511=CARTESIAN_POINT ( 'NONE',  ( 8.426051298355536900, 4.623896040499394289, 154.5496813259660769 ) ) ;
#37531=EDGE_CURVE ( 'NONE', #32027, #18459, #24724, .T. ) ;
#37559=ORIENTED_EDGE ( 'NONE', *, *, #2193, .F. ) ;
#37572=ORIENTED_EDGE ( 'NONE', *, *, #5785, .T. ) ;
#37575=ORIENTED_EDGE ( 'NONE', *, *, #36254, .F. ) ;
#37580=DIRECTION ( 'NONE',  ( -1.000000000000000000, 0.000000000000000000, 0.000000000000000000 ) ) ;
#37583=DIRECTION ( 'NONE',  ( -1.000000000000000000, 0.000000000000000000, 0.000000000000000000 ) ) ;
#37637=ADVANCED_FACE ( 'NONE', ( #23001 ), #23210, .F. ) ;
#37656=EDGE_CURVE ( 'NONE', #32814, #2257, #39363, .T. ) ;
#37663=DIRECTION ( 'NONE',  ( -1.000000000000000000, 0.000000000000000000, 0.000000000000000000 ) ) ;
#37666=CARTESIAN_POINT ( 'NONE',  ( 16.28249153430138207, 8.099299129593287461, 159.5815388724490163 ) ) ;
#37677=CIRCLE ( 'NONE', #19331, 11.07917404492548030 ) ;
#37682=VERTEX_POINT ( 'NONE', #20453 ) ;
#37683=CARTESIAN_POINT ( 'NONE',  ( 1.196959198423996895E-13, 12.49999999999998401, 159.5815388724490163 ) ) ;
#37706=LINE ( 'NONE', #18343, #15110 ) ;
#37721=ORIENTED_EDGE ( 'NONE', *, *, #34418, .F. ) ;
#37735=ORIENTED_EDGE ( 'NONE', *, *, #41854, .T. ) ;
#37743=DIRECTION ( 'NONE',  ( 1.000000000000000000, 0.000000000000000000, 0.000000000000000000 ) ) ;
#37748=DIRECTION ( 'NONE',  ( -0.000000000000000000, -0.000000000000000000, -1.000000000000000000 ) ) ;
#37773=CARTESIAN_POINT ( 'NONE',  ( 0.000000000000000000, 17.49999999999998934, 150.5815388724490163 ) ) ;
#37812=EDGE_LOOP ( 'NONE', ( #36146, #2421, #37559, #15301 ) ) ;
#37814=CARTESIAN_POINT ( 'NONE',  ( 8.536601555665292551, 27.62022878026183292, 153.2247034666966101 ) ) ;
#37830=CARTESIAN_POINT ( 'NONE',  ( 1.263023857913728065, 6.178495204265140650, 152.0797566321136856 ) ) ;
#37835=SPHERICAL_SURFACE ( 'NONE', #24899, 5.000000000000000000 ) ;
#37839=DIRECTION ( 'NONE',  ( -1.000000000000000000, 0.000000000000000000, -0.000000000000000000 ) ) ;
#37842=VERTEX_POINT ( 'NONE', #18096 ) ;
#37881=EDGE_CURVE ( 'NONE', #2257, #1623, #31474, .T. ) ;
#37892=VERTEX_POINT ( 'NONE', #40843 ) ;
#37899=ADVANCED_FACE ( 'NONE', ( #32321 ), #15746, .T. ) ;
#37901=AXIS2_PLACEMENT_3D ( 'NONE', #24533, #37499, #31115 ) ;
#37916=VERTEX_POINT ( 'NONE', #12545 ) ;
#37941=VERTEX_POINT ( 'NONE', #34881 ) ;
#37992=AXIS2_PLACEMENT_3D ( 'NONE', #37238, #8092, #21070 ) ;
#37994=AXIS2_PLACEMENT_3D ( 'NONE', #14579, #27554, #33725 ) ;
#38007=ORIENTED_EDGE ( 'NONE', *, *, #24877, .T. ) ;
#38024=VECTOR ( 'NONE', #23245, 1000.000000000000000 ) ;
#38028=CARTESIAN_POINT ( 'NONE',  ( 0.000000000000000000, 36.30140174081339666, 159.5815388724490163 ) ) ;
#38040=EDGE_CURVE ( 'NONE', #4262, #8699, #19277, .T. ) ;
#38059=CARTESIAN_POINT ( 'NONE',  ( 10.41947860041720908, 17.49999999999956302, 159.5815388724490163 ) ) ;
#38063=VECTOR ( 'NONE', #11394, 1000.000000000000000 ) ;
#38064=CARTESIAN_POINT ( 'NONE',  ( 7.786277848953321978, 6.102744708772449123, 153.5727845928847444 ) ) ;
#38078=VERTEX_POINT ( 'NONE', #10832 ) ;
#38111=VECTOR ( 'NONE', #38584, 1000.000000000000000 ) ;
#38120=DIRECTION ( 'NONE',  ( -0.000000000000000000, 0.000000000000000000, 1.000000000000000000 ) ) ;
#38123=DIRECTION ( 'NONE',  ( -0.000000000000000000, 0.000000000000000000, 1.000000000000000000 ) ) ;
#38131=CARTESIAN_POINT ( 'NONE',  ( -10.20684115509165224, 8.306252114835197986, 150.5815388724490163 ) ) ;
#38146=ORIENTED_EDGE ( 'NONE', *, *, #32452, .T. ) ;
#38150=ORIENTED_EDGE ( 'NONE', *, *, #30448, .F. ) ;
#38154=PLANE ( 'NONE',  #3429 ) ;
#38185=ADVANCED_FACE ( 'NONE', ( #34211 ), #24651, .F. ) ;
#38193=ORIENTED_EDGE ( 'NONE', *, *, #10909, .F. ) ;
#38220=LINE ( 'NONE', #9081, #40408 ) ;
#38223=DIRECTION ( 'NONE',  ( 0.000000000000000000, -0.000000000000000000, -1.000000000000000000 ) ) ;
#38265=DIRECTION ( 'NONE',  ( -0.8485019580238707393, 0.5291922403339430758, -0.000000000000000000 ) ) ;
#38278=DIRECTION ( 'NONE',  ( -1.000000000000000000, 0.000000000000000000, 0.000000000000000000 ) ) ;
#38308=EDGE_LOOP ( 'NONE', ( #30995, #26484, #15370, #3612 ) ) ;
#38330=AXIS2_PLACEMENT_3D ( 'NONE', #29056, #26093, #9934 ) ;
#38347=CARTESIAN_POINT ( 'NONE',  ( 8.886277873992881382, 5.080910142698555454, 154.4799523825326162 ) ) ;
#38351=ADVANCED_FACE ( 'NONE', ( #15070 ), #8059, .T. ) ;
#38359=CARTESIAN_POINT ( 'NONE',  ( 13.91947860041720908, 17.49999999999956302, 153.6452861111154675 ) ) ;
#38368=CIRCLE ( 'NONE', #40407, 5.000000000000000888 ) ;
#38405=( GEOMETRIC_REPRESENTATION_CONTEXT ( 3 ) GLOBAL_UNCERTAINTY_ASSIGNED_CONTEXT ( ( #16932 ) ) GLOBAL_UNIT_ASSIGNED_CONTEXT ( ( #11327, #17923, #14741 ) ) REPRESENTATION_CONTEXT ( 'NONE', 'WORKASPACE' ) );
#38421=VERTEX_POINT ( 'NONE', #21861 ) ;
#38422=CARTESIAN_POINT ( 'NONE',  ( -14.29598715238397055, 14.33504760160264446, 154.0913466422288423 ) ) ;
#38458=DIRECTION ( 'NONE',  ( -1.000000000000000000, 0.000000000000000000, 0.000000000000000000 ) ) ;
#38462=CARTESIAN_POINT ( 'NONE',  ( -2.173728193257111752, 29.03396453015105294, 152.2937014792875914 ) ) ;
#38464=EDGE_LOOP ( 'NONE', ( #17487, #34589, #20471, #27380 ) ) ;
#38469=ORIENTED_EDGE ( 'NONE', *, *, #29359, .F. ) ;
#38563=CARTESIAN_POINT ( 'NONE',  ( -16.28249153430137852, 26.90070087040669478, 159.5815388724490163 ) ) ;
#38584=DIRECTION ( 'NONE',  ( -0.000000000000000000, -0.000000000000000000, -1.000000000000000000 ) ) ;
#38641=FACE_OUTER_BOUND ( 'NONE', #9364, .T. ) ;
#38666=CARTESIAN_POINT ( 'NONE',  ( -3.596493781833085990, 31.27413757694067797, 153.8381731320195911 ) ) ;
#38669=CARTESIAN_POINT ( 'NONE',  ( -5.530144355238147291, 4.987939254928901001, 153.4965619403753010 ) ) ;
#38671=FACE_OUTER_BOUND ( 'NONE', #5032, .T. ) ;
#38673=ORIENTED_EDGE ( 'NONE', *, *, #1693, .F. ) ;
#38675=DIRECTION ( 'NONE',  ( 0.000000000000000000, 0.000000000000000000, -1.000000000000000000 ) ) ;
#38678=CARTESIAN_POINT ( 'NONE',  ( 13.53301942716741024, 15.89449707249891297, 153.4645911160907588 ) ) ;
#38693=B_SPLINE_CURVE_WITH_KNOTS ( 'NONE', 3,
 ( #41448, #31861, #24869, #15080, #2731, #15934, #41026, #15715, #11877, #37830, #28668, #21658, #18476, #9329, #35269, #6129 ),
 .UNSPECIFIED., .F., .F.,
 ( 4, 2, 2, 2, 2, 2, 2, 4 ),
 ( 2.442785351361871688E-07, 0.001910986702701401993, 0.002866357914784545789, 0.003821729126867688935, 0.004777100338950832081, 0.005732471551033974794, 0.006687842763117117506, 0.007643213975200260218 ),
 .UNSPECIFIED. ) ;
#38712=ORIENTED_EDGE ( 'NONE', *, *, #19738, .T. ) ;
#38746=DIRECTION ( 'NONE',  ( 0.000000000000000000, -1.000000000000000000, 0.000000000000000000 ) ) ;
#38748=AXIS2_PLACEMENT_3D ( 'NONE', #38563, #58, #35587 ) ;
#38752=DIRECTION ( 'NONE',  ( 1.000000000000000000, 0.000000000000000000, 0.000000000000000000 ) ) ;
#38773=CIRCLE ( 'NONE', #9567, 4.999999999999999112 ) ;
#38847=FACE_OUTER_BOUND ( 'NONE', #17596, .T. ) ;
#38859=CARTESIAN_POINT ( 'NONE',  ( -13.38682700280587845, 19.36188603005023978, 153.3951907928779974 ) ) ;
#38876=CARTESIAN_POINT ( 'NONE',  ( -6.303637636350195805, 31.40714349395856786, 154.4788437011418125 ) ) ;
#38879=CARTESIAN_POINT ( 'NONE',  ( -8.158171636104116331, 6.584783003016896785, 153.4640812521339797 ) ) ;
#38897=DIRECTION ( 'NONE',  ( -0.000000000000000000, -0.000000000000000000, -1.000000000000000000 ) ) ;
#38936=CARTESIAN_POINT ( 'NONE',  ( -2.604869650104253420, 31.41246745148119857, 159.5815388724490163 ) ) ;
#38980=CARTESIAN_POINT ( 'NONE',  ( 10.20684115509065926, 26.69374788516359942, 153.5324451153148573 ) ) ;
#38995=CIRCLE ( 'NONE', #13890, 11.07917404492619795 ) ;
#39013=DIRECTION ( 'NONE',  ( -0.000000000000000000, -0.000000000000000000, -1.000000000000000000 ) ) ;
#39020=CARTESIAN_POINT ( 'NONE',  ( 0.000000000000000000, 17.49999999999998934, 159.5815388724490163 ) ) ;
#39024=VECTOR ( 'NONE', #40164, 1000.000000000000000 ) ;
#39037=DIRECTION ( 'NONE',  ( 0.8485019580238936099, 0.5291922403339062164, 0.000000000000000000 ) ) ;
#39063=CARTESIAN_POINT ( 'NONE',  ( -13.12940535518774787, 19.71989224933289364, 153.2716026109637255 ) ) ;
#39073=CIRCLE ( 'NONE', #35007, 6.079174044926197951 ) ;
#39109=EDGE_CURVE ( 'NONE', #21748, #7487, #14555, .T. ) ;
#39155=CARTESIAN_POINT ( 'NONE',  ( 9.555006584822203664, 11.60455934013308266, 151.9779333824603782 ) ) ;
#39204=CARTESIAN_POINT ( 'NONE',  ( -10.20684115509089729, 26.69374788516367758, 150.5815388724490163 ) ) ;
#39283=DIRECTION ( 'NONE',  ( -0.000000000000000000, -0.000000000000000000, -1.000000000000000000 ) ) ;
#39297=AXIS2_PLACEMENT_3D ( 'NONE', #22031, #5868, #31799 ) ;
#39323=CARTESIAN_POINT ( 'NONE',  ( 2.429273991871168104, 30.72337055623773949, 153.3506918668360868 ) ) ;
#39335=CARTESIAN_POINT ( 'NONE',  ( -15.41947860041774376, 17.93728447096053458, 154.5727510624246861 ) ) ;
#39359=VECTOR ( 'NONE', #7752, 1000.000000000000000 ) ;
#39363=LINE ( 'NONE', #14076, #8399 ) ;
#39392=CARTESIAN_POINT ( 'NONE',  ( -10.58177606127862802, 24.77416423458351602, 152.9768715113188762 ) ) ;
#39422=VECTOR ( 'NONE', #2608, 1000.000000000000000 ) ;
#39434=CARTESIAN_POINT ( 'NONE',  ( -13.71362260573169678, 16.30792630674986299, 153.5495167475181972 ) ) ;
#39445=CARTESIAN_POINT ( 'NONE',  ( 12.27165144158600185, 20.46975685308311554, 152.8454421597756436 ) ) ;
#39478=CARTESIAN_POINT ( 'NONE',  ( 15.41947860041720908, 17.49999999999956302, 154.5727510624243166 ) ) ;
#39479=CARTESIAN_POINT ( 'NONE',  ( -13.59845369259879888, 18.97199050701624401, 153.4954411043904940 ) ) ;
#39495=CARTESIAN_POINT ( 'NONE',  ( -6.089894672131331177, 31.45012083629602984, 154.4494414891310896 ) ) ;
#39506=ORIENTED_EDGE ( 'NONE', *, *, #39719, .T. ) ;
#39540=CARTESIAN_POINT ( 'NONE',  ( 1.737309318839871608, 30.47044131867540884, 153.1288291135476243 ) ) ;
#39550=ORIENTED_EDGE ( 'NONE', *, *, #39109, .F. ) ;
#39569=AXIS2_PLACEMENT_3D ( 'NONE', #24262, #17874, #40619 ) ;
#39570=CARTESIAN_POINT ( 'NONE',  ( -10.41947860041774199, 17.49999999999951683, 159.5815388724490163 ) ) ;
#39571=LINE ( 'NONE', #23640, #12325 ) ;
#39586=CARTESIAN_POINT ( 'NONE',  ( -4.826850757002720371, 3.486703980550894144, 154.2021328595034220 ) ) ;
#39592=DIRECTION ( 'NONE',  ( 0.8660254037844328234, 0.5000000000000101030, 0.000000000000000000 ) ) ;
#39594=ORIENTED_EDGE ( 'NONE', *, *, #12255, .F. ) ;
#39600=CARTESIAN_POINT ( 'NONE',  ( -5.209739300208506840, 26.52353316214900047, 159.5815388724490163 ) ) ;
#39635=CARTESIAN_POINT ( 'NONE',  ( -11.28496987124454520, 11.56990314725361735, 152.9195735306845734 ) ) ;
#39688=CARTESIAN_POINT ( 'NONE',  ( 1.196959198423996895E-13, 6.277772304111523205, 159.5815388724490163 ) ) ;
#39689=FACE_OUTER_BOUND ( 'NONE', #38464, .T. ) ;
#39693=CARTESIAN_POINT ( 'NONE',  ( 13.06543980208709499, 13.25749020988031823, 153.5324451153150562 ) ) ;
#39694=CARTESIAN_POINT ( 'NONE',  ( -13.53301942716789164, 19.10550292750027523, 153.4645911160910998 ) ) ;
#39714=EDGE_CURVE ( 'NONE', #4671, #2682, #10567, .T. ) ;
#39719=EDGE_CURVE ( 'NONE', #37682, #36157, #8765, .T. ) ;
#39731=EDGE_CURVE ( 'NONE', #15172, #14462, #10141, .T. ) ;
#39738=VECTOR ( 'NONE', #21524, 1000.000000000000000 ) ;
#39764=CARTESIAN_POINT ( 'NONE',  ( -2.437533878364124273, 30.71191045119945429, 153.3425884160443502 ) ) ;
#39802=CARTESIAN_POINT ( 'NONE',  ( 8.815590319779332162, 9.540874024169918144, 152.3738871122218086 ) ) ;
#39817=CARTESIAN_POINT ( 'NONE',  ( 3.813105931423393713, 29.74519779738820802, 152.9676766465810545 ) ) ;
#39836=DIRECTION ( 'NONE',  ( 1.000000000000000000, 1.722326787030199124E-15, 0.000000000000000000 ) ) ;
#39871=ORIENTED_EDGE ( 'NONE', *, *, #40040, .T. ) ;
#39879=DIRECTION ( 'NONE',  ( 1.000000000000000000, 0.000000000000000000, 0.000000000000000000 ) ) ;
#39884=EDGE_CURVE ( 'NONE', #18422, #18459, #3962, .T. ) ;
#39894=CARTESIAN_POINT ( 'NONE',  ( 3.563940842959894884, 5.387559678655692963, 159.5815388724490163 ) ) ;
#39975=DIRECTION ( 'NONE',  ( -0.8660254037844432595, 0.4999999999999919509, 0.000000000000000000 ) ) ;
#40023=CYLINDRICAL_SURFACE ( 'NONE', #30559, 5.000000000000000000 ) ;
#40040=EDGE_CURVE ( 'NONE', #27989, #2489, #19594, .T. ) ;
#40064=CARTESIAN_POINT ( 'NONE',  ( -12.86284886260908777, 13.13113864154247068, 153.4374325591897730 ) ) ;
#40085=ORIENTED_EDGE ( 'NONE', *, *, #28041, .F. ) ;
#40090=CARTESIAN_POINT ( 'NONE',  ( 0.000000000000000000, 17.49999999999998934, 141.5815388724490163 ) ) ;
#40091=VERTEX_POINT ( 'NONE', #12172 ) ;
#40120=DIRECTION ( 'NONE',  ( -0.4702281306424686558, 0.8825449026267667696, 0.000000000000000000 ) ) ;
#40121=VERTEX_POINT ( 'NONE', #19398 ) ;
#40138=CARTESIAN_POINT ( 'NONE',  ( -8.653841190006330564, 27.20987352621967048, 153.0794454334388206 ) ) ;
#40159=EDGE_CURVE ( 'NONE', #18459, #2576, #8985, .T. ) ;
#40164=DIRECTION ( 'NONE',  ( -0.000000000000000000, -0.000000000000000000, -1.000000000000000000 ) ) ;
#40168=CARTESIAN_POINT ( 'NONE',  ( 5.209739300208269697, 26.52353316214887613, 159.5815388724490163 ) ) ;
#40176=DIRECTION ( 'NONE',  ( 1.000000000000000000, 0.000000000000000000, 0.000000000000000000 ) ) ;
#40183=DIRECTION ( 'NONE',  ( 0.000000000000000000, 0.000000000000000000, -1.000000000000000000 ) ) ;
#40228=CARTESIAN_POINT ( 'NONE',  ( -5.463316799720639771, 3.478415450404938714, 154.3424624008201249 ) ) ;
#40230=DIRECTION ( 'NONE',  ( -1.000000000000000000, 0.000000000000000000, 0.000000000000000000 ) ) ;
#40231=VECTOR ( 'NONE', #15218, 1000.000000000000000 ) ;
#40233=ORIENTED_EDGE ( 'NONE', *, *, #1277, .F. ) ;
#40235=DIRECTION ( 'NONE',  ( 0.000000000000000000, 0.000000000000000000, -1.000000000000000000 ) ) ;
#40249=CARTESIAN_POINT ( 'NONE',  ( -12.28238916904392752, 22.29575996873193588, 153.1863241608644444 ) ) ;
#40255=CARTESIAN_POINT ( 'NONE',  ( -10.41947860041774199, 17.49999999999951683, 159.5815388724490163 ) ) ;
#40286=CIRCLE ( 'NONE', #31442, 3.500000000000003997 ) ;
#40289=VECTOR ( 'NONE', #23462, 1000.000000000000000 ) ;
#40315=VECTOR ( 'NONE', #41633, 1000.000000000000000 ) ;
#40327=LINE ( 'NONE', #33940, #21204 ) ;
#40350=CIRCLE ( 'NONE', #14543, 7.579174044924941178 ) ;
#40356=VERTEX_POINT ( 'NONE', #34962 ) ;
#40397=CARTESIAN_POINT ( 'NONE',  ( 1.578877475747889614, 28.88195139703387682, 152.1415020100055813 ) ) ;
#40399=DIRECTION ( 'NONE',  ( 0.000000000000000000, -0.000000000000000000, 1.000000000000000000 ) ) ;
#40407=AXIS2_PLACEMENT_3D ( 'NONE', #29521, #387, #34756 ) ;
#40408=VECTOR ( 'NONE', #28643, 1000.000000000000000 ) ;
#40412=EDGE_LOOP ( 'NONE', ( #40755, #27742, #10692 ) ) ;
#40413=EDGE_CURVE ( 'NONE', #1168, #4147, #9656, .T. ) ;
#40427=AXIS2_PLACEMENT_3D ( 'NONE', #1181, #14149, #973 ) ;
#40436=CARTESIAN_POINT ( 'NONE',  ( -9.724190303530583890, 6.316858655413700951, 154.2011257354768929 ) ) ;
#40442=AXIS2_PLACEMENT_3D ( 'NONE', #11131, #24112, #36650 ) ;
#40472=CIRCLE ( 'NONE', #30295, 5.000000000000004441 ) ;
#40527=CARTESIAN_POINT ( 'NONE',  ( -3.563940842959838040, 29.61244032134267101, 159.5815388724490163 ) ) ;
#40549=CARTESIAN_POINT ( 'NONE',  ( -3.563940842959838040, 29.61244032134267101, 159.5815388724490163 ) ) ;
#40558=DIRECTION ( 'NONE',  ( -0.000000000000000000, -0.000000000000000000, -1.000000000000000000 ) ) ;
#40608=DIRECTION ( 'NONE',  ( 0.000000000000000000, 0.000000000000000000, -1.000000000000000000 ) ) ;
#40619=DIRECTION ( 'NONE',  ( 0.9994203709764837296, -0.03404294460277318413, 0.000000000000000000 ) ) ;
#40645=ORIENTED_EDGE ( 'NONE', *, *, #34230, .T. ) ;
#40651=CARTESIAN_POINT ( 'NONE',  ( 5.209739300208269697, 26.52353316214887613, 164.5815388724490163 ) ) ;
#40653=EDGE_CURVE ( 'NONE', #1623, #28523, #37677, .T. ) ;
#40655=CARTESIAN_POINT ( 'NONE',  ( 0.000000000000000000, 17.49999999999998934, 141.5815388724490163 ) ) ;
#40690=CARTESIAN_POINT ( 'NONE',  ( -3.742640687119191512, 14.18448485343225585, 159.5815388724490163 ) ) ;
#40694=FACE_OUTER_BOUND ( 'NONE', #10637, .T. ) ;
#40696=CARTESIAN_POINT ( 'NONE',  ( 5.665064099548795973, 3.492631074414731085, 154.3802602213502269 ) ) ;
#40700=CARTESIAN_POINT ( 'NONE',  ( 5.000000000000004441, 17.49999999999998934, 159.5815388724490163 ) ) ;
#40701=EDGE_CURVE ( 'NONE', #30300, #7452, #17315, .T. ) ;
#40718=VECTOR ( 'NONE', #30578, 1000.000000000000000 ) ;
#40727=EDGE_CURVE ( 'NONE', #19992, #13358, #15281, .T. ) ;
#40740=AXIS2_PLACEMENT_3D ( 'NONE', #8364, #6438, #16435 ) ;
#40755=ORIENTED_EDGE ( 'NONE', *, *, #31697, .F. ) ;
#40758=ORIENTED_EDGE ( 'NONE', *, *, #36015, .F. ) ;
#40836=CARTESIAN_POINT ( 'NONE',  ( 8.486615222244772383, 7.238047266683384606, 153.2720929549184348 ) ) ;
#40843=CARTESIAN_POINT ( 'NONE',  ( 13.06543980208709677, 13.25749020988032179, 159.5815388724490163 ) ) ;
#40850=CARTESIAN_POINT ( 'NONE',  ( 5.209739300208269697, 26.52353316214887613, 150.5815388724490163 ) ) ;
#40853=DIRECTION ( 'NONE',  ( -0.000000000000000000, -0.000000000000000000, -1.000000000000000000 ) ) ;
#40867=ORIENTED_EDGE ( 'NONE', *, *, #14283, .T. ) ;
#40907=DIRECTION ( 'NONE',  ( 0.000000000000000000, 0.000000000000000000, 1.000000000000000000 ) ) ;
#40912=VECTOR ( 'NONE', #36606, 1000.000000000000000 ) ;
#40916=AXIS2_PLACEMENT_3D ( 'NONE', #27589, #40558, #14406 ) ;
#40920=AXIS2_PLACEMENT_3D ( 'NONE', #30512, #14356, #33916 ) ;
#40939=EDGE_CURVE ( 'NONE', #29296, #27989, #24513, .T. ) ;
#40954=AXIS2_PLACEMENT_3D ( 'NONE', #11465, #40608, #8907 ) ;
#41004=DIRECTION ( 'NONE',  ( 0.000000000000000000, 0.000000000000000000, -1.000000000000000000 ) ) ;
#41008=CARTESIAN_POINT ( 'NONE',  ( 8.698105546966875323, 26.92466507720384072, 152.9675984850764792 ) ) ;
#41026=CARTESIAN_POINT ( 'NONE',  ( -0.3280984336922084799, 6.277401224989384687, 151.9779333920871522 ) ) ;
#41034=ORIENTED_EDGE ( 'NONE', *, *, #6730, .F. ) ;
#41046=LINE ( 'NONE', #41470, #16412 ) ;
#41049=CARTESIAN_POINT ( 'NONE',  ( 6.408084924487494227, 5.174138182523970286, 153.6264000693448963 ) ) ;
#41065=ORIENTED_EDGE ( 'NONE', *, *, #30025, .T. ) ;
#41081=AXIS2_PLACEMENT_3D ( 'NONE', #40255, #6864, #13670 ) ;
#41102=EDGE_CURVE ( 'NONE', #19996, #1168, #28864, .T. ) ;
#41112=LINE ( 'NONE', #14953, #29525 ) ;
#41136=ORIENTED_EDGE ( 'NONE', *, *, #7991, .F. ) ;
#41142=CARTESIAN_POINT ( 'NONE',  ( 13.91947860041720908, 17.80713289880430850, 153.6452861111154959 ) ) ;
#41210=EDGE_LOOP ( 'NONE', ( #35700, #28047, #15937, #225 ) ) ;
#41231=CARTESIAN_POINT ( 'NONE',  ( 0.000000000000000000, 17.49999999999998934, 155.5815388724490163 ) ) ;
#41262=CARTESIAN_POINT ( 'NONE',  ( 5.819810511208063808, 5.026772754302591295, 153.5487751394679776 ) ) ;
#41286=DIRECTION ( 'NONE',  ( -0.000000000000000000, -0.000000000000000000, -1.000000000000000000 ) ) ;
#41287=ORIENTED_EDGE ( 'NONE', *, *, #41102, .F. ) ;
#41293=ORIENTED_EDGE ( 'NONE', *, *, #5140, .T. ) ;
#41328=CARTESIAN_POINT ( 'NONE',  ( -15.15544456622756364, 8.749999999999817035, 154.5815388724490163 ) ) ;
#41342=EDGE_LOOP ( 'NONE', ( #8811, #37572, #22126, #41293 ) ) ;
#41362=ADVANCED_FACE ( 'NONE', ( #31042 ), #21465, .T. ) ;
#41374=CARTESIAN_POINT ( 'NONE',  ( -4.742640687119331844, 19.08346433899860273, 159.5815388724490163 ) ) ;
#41402=ORIENTED_EDGE ( 'NONE', *, *, #32928, .T. ) ;
#41423=DIRECTION ( 'NONE',  ( -0.000000000000000000, 0.000000000000000000, -1.000000000000000000 ) ) ;
#41448=CARTESIAN_POINT ( 'NONE',  ( -3.563940842960075184, 5.387559678655594375, 152.8454421597761552 ) ) ;
#41469=DIRECTION ( 'NONE',  ( 0.5291922403339428538, 0.8485019580238706283, 0.000000000000000000 ) ) ;
#41470=CARTESIAN_POINT ( 'NONE',  ( -13.06543980208746270, 13.25749020988016547, 150.5815388724490163 ) ) ;
#41484=CARTESIAN_POINT ( 'NONE',  ( 16.28249153430137852, 26.90070087040669122, 159.5815388724490163 ) ) ;
#41499=CARTESIAN_POINT ( 'NONE',  ( -4.330127018922123483, 14.99999999999985789, 155.5815388724490163 ) ) ;
#41500=ORIENTED_EDGE ( 'NONE', *, *, #3854, .T. ) ;
#41547=CARTESIAN_POINT ( 'NONE',  ( 4.405423949752161228, 3.537109377885448325, 154.0908813598610152 ) ) ;
#41560=CARTESIAN_POINT ( 'NONE',  ( 13.71362260573116032, 18.69207369324923462, 153.5495167475178562 ) ) ;
#41601=AXIS2_PLACEMENT_3D ( 'NONE', #34320, #15176, #34526 ) ;
#41606=EDGE_LOOP ( 'NONE', ( #27065, #39550 ) ) ;
#41629=EDGE_CURVE ( 'NONE', #17600, #38078, #38368, .T. ) ;
#41633=DIRECTION ( 'NONE',  ( 0.000000000000000000, 0.000000000000000000, 1.000000000000000000 ) ) ;
#41659=CARTESIAN_POINT ( 'NONE',  ( -4.932408324001532840, 30.01561855534181333, 153.3561522493810685 ) ) ;
#41665=VERTEX_POINT ( 'NONE', #2638 ) ;
#41667=DIRECTION ( 'NONE',  ( 0.8660254037844432595, -0.4999999999999919509, 0.000000000000000000 ) ) ;
#41680=CARTESIAN_POINT ( 'NONE',  ( -2.858598646996056036, 30.93625767528277848, 150.5815388724490163 ) ) ;
#41688=AXIS2_PLACEMENT_3D ( 'NONE', #839, #32730, #7431 ) ;
#41726=ORIENTED_EDGE ( 'NONE', *, *, #27531, .T. ) ;
#41737=CARTESIAN_POINT ( 'NONE',  ( 0.000000000000000000, 17.49999999999998934, 154.5815388724490163 ) ) ;
#41793=CARTESIAN_POINT ( 'NONE',  ( -13.06543980208727262, 21.74250979011898721, 159.5815388724490163 ) ) ;
#41809=ORIENTED_EDGE ( 'NONE', *, *, #33968, .T. ) ;
#41812=CIRCLE ( 'NONE', #10556, 6.079174044925164111 ) ;
#41833=CARTESIAN_POINT ( 'NONE',  ( -10.53587323178440194, 22.42818870813906429, 159.5815388724490163 ) ) ;
#41854=EDGE_CURVE ( 'NONE', #13719, #3564, #4638, .T. ) ;
#41870=CYLINDRICAL_SURFACE ( 'NONE', #2883, 5.000000000000004441 ) ;
#41876=CARTESIAN_POINT ( 'NONE',  ( -3.032103446742963282, 29.34858651153008680, 152.5993403105693744 ) ) ;
#41878=CARTESIAN_POINT ( 'NONE',  ( -8.070690082935801257, 28.54527614739936681, 153.4965620064455436 ) ) ;
#41886=FACE_OUTER_BOUND ( 'NONE', #13995, .T. ) ;
#41894=CARTESIAN_POINT ( 'NONE',  ( 9.889506012869997420, 28.29665438702152258, 154.0908813678212539 ) ) ;
#41926=ORIENTED_EDGE ( 'NONE', *, *, #36224, .F. ) ;
#41977=ORIENTED_EDGE ( 'NONE', *, *, #17306, .T. ) ;
#41980=ORIENTED_EDGE ( 'NONE', *, *, #26765, .T. ) ;
#41989=EDGE_CURVE ( 'NONE', #13300, #5194, #12565, .T. ) ;
#42061=DIRECTION ( 'NONE',  ( 0.8660254037844363761, 0.5000000000000039968, 0.000000000000000000 ) ) ;
#42063=FACE_OUTER_BOUND ( 'NONE', #17647, .T. ) ;
#42068=ORIENTED_EDGE ( 'NONE', *, *, #33598, .T. ) ;
#42077=CARTESIAN_POINT ( 'NONE',  ( -4.197921810176622692, 31.42444391617877386, 154.0304303761505764 ) ) ;
#42082=CARTESIAN_POINT ( 'NONE',  ( -4.501085982074576997, 5.045936893373308862, 153.2263580705401864 ) ) ;
#42089=EDGE_LOOP ( 'NONE', ( #20370, #28336, #36575, #20417 ) ) ;
#42098=AXIS2_PLACEMENT_3D ( 'NONE', #34619, #25484, #2925 ) ;
#42153=COLOUR_RGB('Black',0.12,0.14,0.17);
#42154=FILL_AREA_STYLE_COLOUR('',#42153);
#42155=FILL_AREA_STYLE('',(#42154));
#42156=SURFACE_STYLE_FILL_AREA(#42155);
#42157=SURFACE_SIDE_STYLE('',(#42156));
#42158=SURFACE_STYLE_USAGE(.BOTH.,#42157);
#42159=PRESENTATION_STYLE_ASSIGNMENT((#42158));
ENDSEC;
END-ISO-10303-21;
